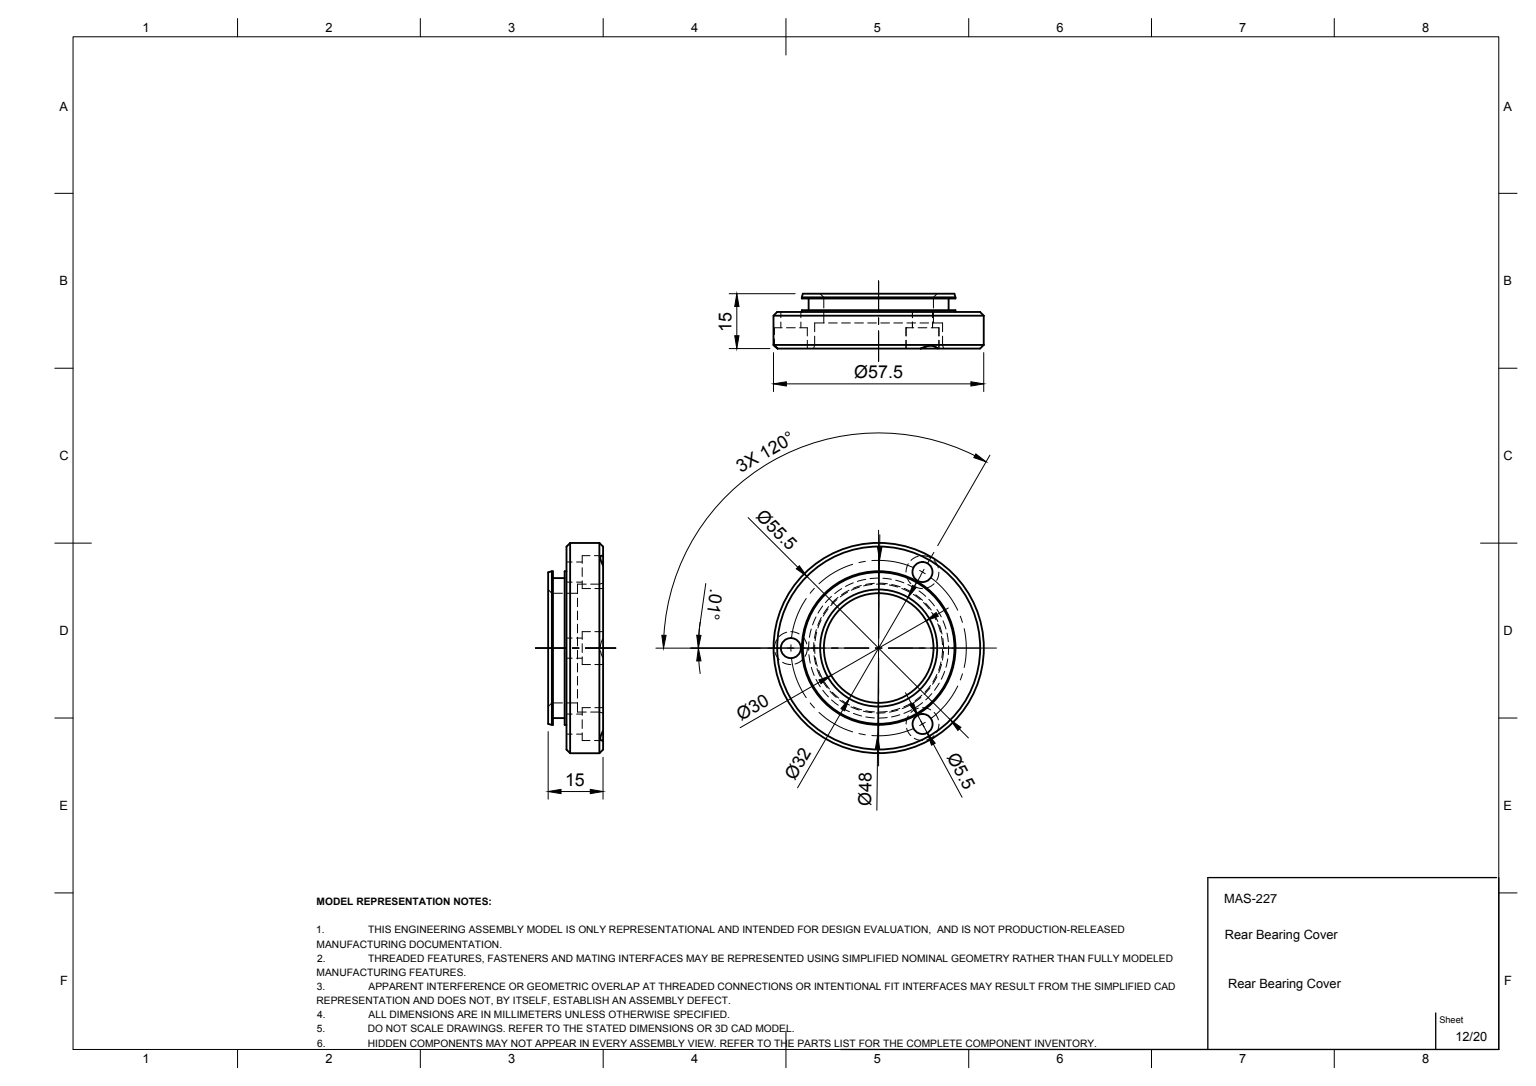
ISO-10303-21;
HEADER;
FILE_DESCRIPTION (('STEP AP214'),
    '1' );
FILE_NAME ( 'Rear Bearing Cover.step', '2026-10-06T08:24:41', ( '' ), ( '' ), 'STEP AP214', 'Unspecified', '' );
FILE_SCHEMA (( 'AUTOMOTIVE_DESIGN' ));
ENDSEC;
DATA;
#7=DIRECTION ( 'NONE',  ( -1.000000000000000000, 0.000000000000000000, 0.000000000000000000 ) ) ;
#24=ORIENTED_EDGE ( 'NONE', *, *, #27873, .F. ) ;
#69=DIRECTION ( 'NONE',  ( 1.000000000000000000, 0.000000000000000000, 0.000000000000000000 ) ) ;
#80=EDGE_LOOP ( 'NONE', ( #10881, #7158 ) ) ;
#89=DIRECTION ( 'NONE',  ( 0.000000000000000000, -1.000000000000000000, 0.000000000000000000 ) ) ;
#102=DIRECTION ( 'NONE',  ( -1.000000000000000000, 0.000000000000000000, 0.000000000000000000 ) ) ;
#208=CARTESIAN_POINT ( 'NONE',  ( -0.01968503937007897581, -0.8214970631411201429, 0.000000000000000000 ) ) ;
#218=VERTEX_POINT ( 'NONE', #1034 ) ;
#239=EDGE_LOOP ( 'NONE', ( #22677, #15160 ) ) ;
#245=DIRECTION ( 'NONE',  ( -1.000000000000000000, 0.000000000000000000, 0.000000000000000000 ) ) ;
#268=ORIENTED_EDGE ( 'NONE', *, *, #11086, .F. ) ;
#315=FACE_OUTER_BOUND ( 'NONE', #4485, .T. ) ;
#445=VECTOR ( 'NONE', #20789, 39.37007874015748854 ) ;
#447=FACE_OUTER_BOUND ( 'NONE', #2356, .T. ) ;
#465=DIRECTION ( 'NONE',  ( 1.000000000000000000, 0.000000000000000000, 0.000000000000000000 ) ) ;
#470=CIRCLE ( 'NONE', #7684, 0.6889763779527560139 ) ;
#587=CIRCLE ( 'NONE', #3254, 0.8267716535433071723 ) ;
#589=ORIENTED_EDGE ( 'NONE', *, *, #19290, .F. ) ;
#648=CARTESIAN_POINT ( 'NONE',  ( -0.01968503937007897581, 0.8214970631411201429, 1.006043748884723849E-16 ) ) ;
#653=DIRECTION ( 'NONE',  ( 0.000000000000000000, -1.000000000000000000, 0.000000000000000000 ) ) ;
#671=DIRECTION ( 'NONE',  ( 0.000000000000000000, -1.000000000000000000, 0.000000000000000000 ) ) ;
#813=DIRECTION ( 'NONE',  ( 1.000000000000000000, 0.000000000000000000, 0.000000000000000000 ) ) ;
#828=ORIENTED_EDGE ( 'NONE', *, *, #19338, .F. ) ;
#844=CIRCLE ( 'NONE', #25418, 0.1771653543307086798 ) ;
#853=CARTESIAN_POINT ( 'NONE',  ( -0.3661417322834645272, -0.4724409448818898127, -0.8182917201112815953 ) ) ;
#863=CYLINDRICAL_SURFACE ( 'NONE', #6726, 0.7539370078740157410 ) ;
#903=ORIENTED_EDGE ( 'NONE', *, *, #16753, .T. ) ;
#912=DIRECTION ( 'NONE',  ( 1.000000000000000000, 0.000000000000000000, 0.000000000000000000 ) ) ;
#919=DIRECTION ( 'NONE',  ( 1.000000000000000000, 0.000000000000000000, 0.000000000000000000 ) ) ;
#989=CARTESIAN_POINT ( 'NONE',  ( -0.3149606299212598381, 0.000000000000000000, 0.000000000000000000 ) ) ;
#1005=ORIENTED_EDGE ( 'NONE', *, *, #22105, .F. ) ;
#1030=CIRCLE ( 'NONE', #19050, 0.8162224727389330026 ) ;
#1034=CARTESIAN_POINT ( 'NONE',  ( -0.5905511811023621549, 0.6995255587508188988, 8.566717364459539934E-17 ) ) ;
#1053=CIRCLE ( 'NONE', #16846, 0.1082677165354330312 ) ;
#1091=ORIENTED_EDGE ( 'NONE', *, *, #9443, .F. ) ;
#1121=ORIENTED_EDGE ( 'NONE', *, *, #6645, .T. ) ;
#1143=CIRCLE ( 'NONE', #10607, 0.1082677165354330312 ) ;
#1159=CARTESIAN_POINT ( 'NONE',  ( -0.1968503937007874127, 0.000000000000000000, 0.000000000000000000 ) ) ;
#1234=DIRECTION ( 'NONE',  ( -1.000000000000000000, 0.000000000000000000, 0.000000000000000000 ) ) ;
#1254=DIRECTION ( 'NONE',  ( 1.000000000000000000, 0.000000000000000000, 0.000000000000000000 ) ) ;
#1287=CARTESIAN_POINT ( 'NONE',  ( -0.1771653543307086520, 0.000000000000000000, 0.000000000000000000 ) ) ;
#1312=SURFACE_SIDE_STYLE ('',( #11903 ) ) ;
#1384=CARTESIAN_POINT ( 'NONE',  ( 2.664928230027803213, 0.9448818897637796255, -1.639108661417322569E-17 ) ) ;
#1398=CARTESIAN_POINT ( 'NONE',  ( -0.5811915241081616612, -0.4724399524670138684, 0.9954595399565421276 ) ) ;
#1402=PLANE ( 'NONE',  #15530 ) ;
#1403=AXIS2_PLACEMENT_3D ( 'NONE', #19008, #6721, #21281 ) ;
#1430=DIRECTION ( 'NONE',  ( 0.000000000000000000, -1.000000000000000000, 0.000000000000000000 ) ) ;
#1484=CIRCLE ( 'NONE', #8268, 0.6299212598425196763 ) ;
#1488=DIRECTION ( 'NONE',  ( 0.000000000000000000, 1.000000000000000000, 0.000000000000000000 ) ) ;
#1496=FACE_OUTER_BOUND ( 'NONE', #23490, .T. ) ;
#1544=ORIENTED_EDGE ( 'NONE', *, *, #11001, .F. ) ;
#1548=FACE_OUTER_BOUND ( 'NONE', #9863, .T. ) ;
#1550=DIRECTION ( 'NONE',  ( -1.000000000000000000, 0.000000000000000000, 0.000000000000000000 ) ) ;
#1579=CARTESIAN_POINT ( 'NONE',  ( -0.5708661417322835607, 0.000000000000000000, 0.000000000000000000 ) ) ;
#1596=CARTESIAN_POINT ( 'NONE',  ( -0.5609636804891235951, -0.5548708868579311781, 0.9753553170056504795 ) ) ;
#1599=CARTESIAN_POINT ( 'NONE',  ( -0.5622642684307268546, -0.5391005349161613891, -0.9826765462749343927 ) ) ;
#1600=FACE_OUTER_BOUND ( 'NONE', #23729, .T. ) ;
#1624=PLANE ( 'NONE',  #18273 ) ;
#1625=FACE_BOUND ( 'NONE', #12857, .T. ) ;
#1645=FACE_OUTER_BOUND ( 'NONE', #3746, .T. ) ;
#1655=CIRCLE ( 'NONE', #3429, 0.1771653543307086798 ) ;
#1676=AXIS2_PLACEMENT_3D ( 'NONE', #17009, #8543, #17159 ) ;
#1738=CARTESIAN_POINT ( 'NONE',  ( -0.5616991426751372085, -0.5770957586701074282, 0.9615147744167586996 ) ) ;
#1763=FACE_OUTER_BOUND ( 'NONE', #3029, .T. ) ;
#1767=CONICAL_SURFACE ( 'NONE', #12147, 0.6102362204724409711, 0.7853981625000032718 ) ;
#1771=PLANE ( 'NONE',  #16654 ) ;
#1773=DIRECTION ( 'NONE',  ( 0.000000000000000000, 0.000000000000000000, 1.000000000000000000 ) ) ;
#1855=DIRECTION ( 'NONE',  ( -1.000000000000000000, 0.000000000000000000, 0.000000000000000000 ) ) ;
#1882=PRODUCT_DEFINITION ( 'UNKNOWN', '', #26496, #17018 ) ;
#1918=DIRECTION ( 'NONE',  ( -1.000000000000000000, 0.000000000000000000, 0.000000000000000000 ) ) ;
#1935=VERTEX_POINT ( 'NONE', #20033 ) ;
#1979=DIRECTION ( 'NONE',  ( 1.000000000000000000, 0.000000000000000000, 0.000000000000000000 ) ) ;
#1980=AXIS2_PLACEMENT_3D ( 'NONE', #7829, #5567, #26603 ) ;
#1995=ORIENTED_EDGE ( 'NONE', *, *, #12248, .F. ) ;
#2026=LINE ( 'NONE', #12899, #6921 ) ;
#2044=DIRECTION ( 'NONE',  ( 1.000000000000000000, 0.000000000000000000, 0.000000000000000000 ) ) ;
#2049=VERTEX_POINT ( 'NONE', #7046 ) ;
#2062=DIRECTION ( 'NONE',  ( 1.000000000000000000, 0.000000000000000000, 0.000000000000000000 ) ) ;
#2064=PLANE ( 'NONE',  #7665 ) ;
#2079=CARTESIAN_POINT ( 'NONE',  ( -0.5708661417322835607, 1.112204724409448842, -1.362057955744595713E-16 ) ) ;
#2103=EDGE_LOOP ( 'NONE', ( #16313, #11756, #24, #10103 ) ) ;
#2107=CARTESIAN_POINT ( 'NONE',  ( -0.5681815575442429322, 1.113574658101619930, 0.05417226358512977624 ) ) ;
#2114=CARTESIAN_POINT ( 'NONE',  ( -0.05118110236220472370, 0.000000000000000000, 0.000000000000000000 ) ) ;
#2165=ORIENTED_EDGE ( 'NONE', *, *, #5688, .F. ) ;
#2201=FACE_BOUND ( 'NONE', #13567, .T. ) ;
#2222=VERTEX_POINT ( 'NONE', #5776 ) ;
#2224=DIRECTION ( 'NONE',  ( -1.000000000000000000, 0.000000000000000000, 0.000000000000000000 ) ) ;
#2253=DIRECTION ( 'NONE',  ( 1.000000000000000000, 0.000000000000000000, 0.000000000000000000 ) ) ;
#2285=ORIENTED_EDGE ( 'NONE', *, *, #21450, .F. ) ;
#2287=ADVANCED_FACE ( 'NONE', ( #12776 ), #25780, .T. ) ;
#2301=DIRECTION ( 'NONE',  ( 0.000000000000000000, 0.000000000000000000, 1.000000000000000000 ) ) ;
#2302=ADVANCED_FACE ( 'NONE', ( #27767, #15193 ), #1624, .T. ) ;
#2356=EDGE_LOOP ( 'NONE', ( #13538, #26483, #11394, #8210 ) ) ;
#2363=CARTESIAN_POINT ( 'NONE',  ( -0.1968503937007874127, -0.4724409448818898127, 0.8182917201112815953 ) ) ;
#2369=VECTOR ( 'NONE', #13146, 39.37007874015748143 ) ;
#2377=ORIENTED_EDGE ( 'NONE', *, *, #27274, .F. ) ;
#2380=CARTESIAN_POINT ( 'NONE',  ( -2.185478346456693112E-16, 0.000000000000000000, 0.000000000000000000 ) ) ;
#2382=VECTOR ( 'NONE', #13266, 39.37007874015748143 ) ;
#2412=CARTESIAN_POINT ( 'NONE',  ( -0.5511811023622047445, -0.6889763779527560139, 8.437527159479796553E-17 ) ) ;
#2423=DIRECTION ( 'NONE',  ( 1.000000000000000000, 0.000000000000000000, 0.000000000000000000 ) ) ;
#2424=ORIENTED_EDGE ( 'NONE', *, *, #27873, .T. ) ;
#2434=VECTOR ( 'NONE', #8777, 39.37007874015748143 ) ;
#2438=CARTESIAN_POINT ( 'NONE',  ( -0.5708661417322835607, -0.6942509683549429322, 0.000000000000000000 ) ) ;
#2469=CARTESIAN_POINT ( 'NONE',  ( -0.02559055118110236185, 0.000000000000000000, 0.000000000000000000 ) ) ;
#2512=CARTESIAN_POINT ( 'NONE',  ( -0.3661417322834645272, 0.9448818897637796255, -1.639108661417322569E-17 ) ) ;
#2523=CARTESIAN_POINT ( 'NONE',  ( -0.05118110236220472370, 0.7903543307086614567, 0.000000000000000000 ) ) ;
#2528=CARTESIAN_POINT ( 'NONE',  ( -0.1141732283464566844, 0.7539370078740157410, 0.000000000000000000 ) ) ;
#2549=VECTOR ( 'NONE', #10663, 39.37007874015748143 ) ;
#2605=AXIS2_PLACEMENT_3D ( 'NONE', #9872, #10429, #27399 ) ;
#2610=AXIS2_PLACEMENT_3D ( 'NONE', #8395, #23235, #3870 ) ;
#2643=ORIENTED_EDGE ( 'NONE', *, *, #3133, .T. ) ;
#2656=AXIS2_PLACEMENT_3D ( 'NONE', #9060, #23786, #89 ) ;
#2687=DIRECTION ( 'NONE',  ( 0.000000000000000000, -1.000000000000000000, 0.000000000000000000 ) ) ;
#2728=ADVANCED_FACE ( 'NONE', ( #4189 ), #21424, .T. ) ;
#2758=EDGE_LOOP ( 'NONE', ( #12853, #9072, #23845, #6887 ) ) ;
#2760=EDGE_CURVE ( 'NONE', #13081, #6094, #26969, .T. ) ;
#2826=VECTOR ( 'NONE', #2224, 39.37007874015748143 ) ;
#2839=CARTESIAN_POINT ( 'NONE',  ( -0.05118110236220472370, 0.8267716535433071723, 0.000000000000000000 ) ) ;
#2859=CYLINDRICAL_SURFACE ( 'NONE', #19118, 0.8267716535433071723 ) ;
#2860=VECTOR ( 'NONE', #11180, 39.37007874015748143 ) ;
#2904=CONICAL_SURFACE ( 'NONE', #12415, 1.112204724409448842, 0.7853981625000011624 ) ;
#2954=CYLINDRICAL_SURFACE ( 'NONE', #14208, 0.1771653543307086798 ) ;
#2963=ORIENTED_EDGE ( 'NONE', *, *, #26481, .F. ) ;
#3024=CARTESIAN_POINT ( 'NONE',  ( -0.03937007874015747977, 0.000000000000000000, 0.000000000000000000 ) ) ;
#3027=VERTEX_POINT ( 'NONE', #12489 ) ;
#3029=EDGE_LOOP ( 'NONE', ( #11928, #9052, #17562, #5731, #24652 ) ) ;
#3074=EDGE_CURVE ( 'NONE', #14891, #4135, #23792, .T. ) ;
#3080=AXIS2_PLACEMENT_3D ( 'NONE', #20906, #1550, #16814 ) ;
#3109=EDGE_CURVE ( 'NONE', #9597, #14042, #11187, .T. ) ;
#3124=CARTESIAN_POINT ( 'NONE',  ( -0.4783464566929133688, -0.4724409448818898127, -0.8182917201112815953 ) ) ;
#3133=EDGE_CURVE ( 'NONE', #12001, #8922, #22523, .T. ) ;
#3146=LINE ( 'NONE', #11777, #7662 ) ;
#3178=ORIENTED_EDGE ( 'NONE', *, *, #23388, .T. ) ;
#3232=VERTEX_POINT ( 'NONE', #22378 ) ;
#3239=VERTEX_POINT ( 'NONE', #12065 ) ;
#3254=AXIS2_PLACEMENT_3D ( 'NONE', #4997, #919, #13619 ) ;
#3261=DIRECTION ( 'NONE',  ( -1.000000000000000000, 0.000000000000000000, 0.000000000000000000 ) ) ;
#3278=CARTESIAN_POINT ( 'NONE',  ( -0.3149606299212598381, 0.000000000000000000, 0.000000000000000000 ) ) ;
#3293=VERTEX_POINT ( 'NONE', #9801 ) ;
#3312=CARTESIAN_POINT ( 'NONE',  ( -0.03937007874015747977, 0.000000000000000000, 0.000000000000000000 ) ) ;
#3325=EDGE_CURVE ( 'NONE', #25692, #23663, #26075, .T. ) ;
#3357=EDGE_LOOP ( 'NONE', ( #19208, #4870, #20216, #2165 ) ) ;
#3360=UNCERTAINTY_MEASURE_WITH_UNIT (LENGTH_MEASURE( 1.000000000000000082E-05 ), #12173, 'distance_accuracy_value', 'NONE') ;
#3429=AXIS2_PLACEMENT_3D ( 'NONE', #25649, #6303, #23547 ) ;
#3441=ORIENTED_EDGE ( 'NONE', *, *, #26709, .T. ) ;
#3463=DIRECTION ( 'NONE',  ( 0.000000000000000000, -1.000000000000000000, 0.000000000000000000 ) ) ;
#3495=DIRECTION ( 'NONE',  ( -1.000000000000000000, 0.000000000000000000, 0.000000000000000000 ) ) ;
#3516=VECTOR ( 'NONE', #2253, 39.37007874015748143 ) ;
#3534=CARTESIAN_POINT ( 'NONE',  ( -2.185478346456693112E-16, 0.000000000000000000, 0.000000000000000000 ) ) ;
#3537=VECTOR ( 'NONE', #15870, 39.37007874015748143 ) ;
#3546=AXIS2_PLACEMENT_3D ( 'NONE', #17760, #9267, #5182 ) ;
#3575=SHAPE_REPRESENTATION ( 'Rear Bearing Cover', ( #11588 ), #19278 ) ;
#3610=CARTESIAN_POINT ( 'NONE',  ( -0.05118110236220472370, 0.7539370078740157410, 0.000000000000000000 ) ) ;
#3665=DIRECTION ( 'NONE',  ( 0.000000000000000000, 0.000000000000000000, 1.000000000000000000 ) ) ;
#3681=ORIENTED_EDGE ( 'NONE', *, *, #6118, .F. ) ;
#3697=AXIS2_PLACEMENT_3D ( 'NONE', #11160, #17904, #22309 ) ;
#3714=CARTESIAN_POINT ( 'NONE',  ( -0.5616993144963264850, -0.5770964849842729061, -0.9615141454532954990 ) ) ;
#3728=CONICAL_SURFACE ( 'NONE', #24035, 0.8214970631411201429, 0.2617993875000020898 ) ;
#3746=EDGE_LOOP ( 'NONE', ( #23859, #6534 ) ) ;
#3789=ORIENTED_EDGE ( 'NONE', *, *, #4673, .F. ) ;
#3797=EDGE_CURVE ( 'NONE', #16095, #12969, #16768, .T. ) ;
#3800=DIRECTION ( 'NONE',  ( 0.000000000000000000, 0.000000000000000000, 1.000000000000000000 ) ) ;
#3809=DIRECTION ( 'NONE',  ( -1.000000000000000000, 0.000000000000000000, 0.000000000000000000 ) ) ;
#3819=VERTEX_POINT ( 'NONE', #5474 ) ;
#3835=ORIENTED_EDGE ( 'NONE', *, *, #10679, .F. ) ;
#3863=CARTESIAN_POINT ( 'NONE',  ( -0.5819147541874519769, -0.6280848967520352710, -0.9045786101298314286 ) ) ;
#3870=DIRECTION ( 'NONE',  ( 0.000000000000000000, 0.000000000000000000, 1.000000000000000000 ) ) ;
#3887=DIRECTION ( 'NONE',  ( 0.000000000000000000, 0.000000000000000000, 1.000000000000000000 ) ) ;
#3891=ORIENTED_EDGE ( 'NONE', *, *, #11596, .T. ) ;
#3892=VERTEX_POINT ( 'NONE', #24953 ) ;
#3897=ORIENTED_EDGE ( 'NONE', *, *, #14924, .T. ) ;
#3905=CARTESIAN_POINT ( 'NONE',  ( -0.1574803149606299191, 0.000000000000000000, 0.000000000000000000 ) ) ;
#3936=DIRECTION ( 'NONE',  ( 0.000000000000000000, -1.000000000000000000, 0.000000000000000000 ) ) ;
#3942=CARTESIAN_POINT ( 'NONE',  ( -0.4783464566929133688, 0.9448818897637796255, -1.639108661417322569E-17 ) ) ;
#3951=DIRECTION ( 'NONE',  ( 0.000000000000000000, 0.000000000000000000, 1.000000000000000000 ) ) ;
#3973=CARTESIAN_POINT ( 'NONE',  ( -0.5905511811023621549, -0.6348133144914153148, 0.8891632684400255782 ) ) ;
#4008=ADVANCED_FACE ( 'NONE', ( #11441 ), #20198, .F. ) ;
#4012=CARTESIAN_POINT ( 'NONE',  ( -0.3661417322834645272, 0.9448818897637796255, -0.1771653543307086520 ) ) ;
#4025=EDGE_LOOP ( 'NONE', ( #15939, #13089, #26409, #6919 ) ) ;
#4029=ADVANCED_FACE ( 'NONE', ( #16112 ), #863, .T. ) ;
#4036=DIRECTION ( 'NONE',  ( 0.000000000000000000, 0.000000000000000000, 1.000000000000000000 ) ) ;
#4051=CARTESIAN_POINT ( 'NONE',  ( -2.185478346456693112E-16, -0.6299212598071869396, 0.000000000000000000 ) ) ;
#4082=CARTESIAN_POINT ( 'NONE',  ( -0.4783464566929133688, -0.4724409448818898127, -0.8182917201112815953 ) ) ;
#4099=EDGE_CURVE ( 'NONE', #22689, #27836, #10771, .T. ) ;
#4111=DIRECTION ( 'NONE',  ( 0.000000000000000000, 0.000000000000000000, 1.000000000000000000 ) ) ;
#4127=DIRECTION ( 'NONE',  ( -1.000000000000000000, 0.000000000000000000, 0.000000000000000000 ) ) ;
#4135=VERTEX_POINT ( 'NONE', #20026 ) ;
#4139=CARTESIAN_POINT ( 'NONE',  ( 2.664928230027803213, -0.4724409448818898127, -0.9265594366467145848 ) ) ;
#4146=CARTESIAN_POINT ( 'NONE',  ( -0.5608506285916234901, -0.5625436374635495174, -0.9710811323268585538 ) ) ;
#4164=ORIENTED_EDGE ( 'NONE', *, *, #25217, .F. ) ;
#4189=FACE_OUTER_BOUND ( 'NONE', #17127, .T. ) ;
#4190=FACE_OUTER_BOUND ( 'NONE', #26019, .T. ) ;
#4248=DIRECTION ( 'NONE',  ( 1.000000000000000000, 0.000000000000000000, 0.000000000000000000 ) ) ;
#4275=ORIENTED_EDGE ( 'NONE', *, *, #25762, .T. ) ;
#4285=AXIS2_PLACEMENT_3D ( 'NONE', #25571, #8469, #12703 ) ;
#4293=LINE ( 'NONE', #11400, #12043 ) ;
#4334=EDGE_LOOP ( 'NONE', ( #26514, #26729, #27046, #19687 ) ) ;
#4367=CARTESIAN_POINT ( 'NONE',  ( -0.5810616737516007824, 1.098416878720776424, 0.09031125883555725375 ) ) ;
#4384=ORIENTED_EDGE ( 'NONE', *, *, #25655, .T. ) ;
#4441=CIRCLE ( 'NONE', #14833, 0.6889763779527560139 ) ;
#4447=DIRECTION ( 'NONE',  ( 0.000000000000000000, 0.000000000000000000, 1.000000000000000000 ) ) ;
#4451=ORIENTED_EDGE ( 'NONE', *, *, #4099, .F. ) ;
#4463=CARTESIAN_POINT ( 'NONE',  ( -0.3661417322834645272, -0.4724409448818898127, -0.6411263657805729155 ) ) ;
#4485=EDGE_LOOP ( 'NONE', ( #17552, #1995, #17553, #9444 ) ) ;
#4568=APPLICATION_CONTEXT ( 'automotive_design' ) ;
#4589=DIRECTION ( 'NONE',  ( 0.000000000000000000, -1.000000000000000000, 0.000000000000000000 ) ) ;
#4591=EDGE_CURVE ( 'NONE', #14336, #3819, #14026, .T. ) ;
#4599=DIRECTION ( 'NONE',  ( 1.000000000000000000, 0.000000000000000000, 0.000000000000000000 ) ) ;
#4622=DIRECTION ( 'NONE',  ( -1.000000000000000000, 0.000000000000000000, 0.000000000000000000 ) ) ;
#4650=EDGE_CURVE ( 'NONE', #2222, #5851, #10328, .T. ) ;
#4662=DIRECTION ( 'NONE',  ( 0.000000000000000000, 0.000000000000000000, 1.000000000000000000 ) ) ;
#4665=VECTOR ( 'NONE', #13639, 39.37007874015748854 ) ;
#4673=EDGE_CURVE ( 'NONE', #25416, #22409, #21629, .T. ) ;
#4705=CIRCLE ( 'NONE', #24121, 0.7539370078740157410 ) ;
#4712=CARTESIAN_POINT ( 'NONE',  ( 2.664928230027803213, -0.4724409448818898127, 0.9265594366467145848 ) ) ;
#4751=CIRCLE ( 'NONE', #16056, 0.8267716535433071723 ) ;
#4775=ORIENTED_EDGE ( 'NONE', *, *, #23661, .F. ) ;
#4817=CARTESIAN_POINT ( 'NONE',  ( -0.5905511811023621549, 0.000000000000000000, 0.000000000000000000 ) ) ;
#4870=ORIENTED_EDGE ( 'NONE', *, *, #4591, .T. ) ;
#4878=DIRECTION ( 'NONE',  ( 0.7071067818211385081, 0.7071067805519564153, -8.659560554583433905E-17 ) ) ;
#4906=CARTESIAN_POINT ( 'NONE',  ( -0.5610235350335921467, 1.122047331090474165, 0.009609423978176654876 ) ) ;
#4942=ADVANCED_FACE ( 'NONE', ( #20516 ), #26719, .F. ) ;
#4953=EDGE_LOOP ( 'NONE', ( #14615, #22620 ) ) ;
#4968=EDGE_CURVE ( 'NONE', #6094, #25761, #18367, .T. ) ;
#4997=CARTESIAN_POINT ( 'NONE',  ( -0.05118110236220472370, 0.000000000000000000, 0.000000000000000000 ) ) ;
#5023=VERTEX_POINT ( 'NONE', #2839 ) ;
#5035=AXIS2_PLACEMENT_3D ( 'NONE', #23800, #15468, #4447 ) ;
#5059=ORIENTED_EDGE ( 'NONE', *, *, #16111, .T. ) ;
#5109=CONICAL_SURFACE ( 'NONE', #26758, 0.8214970631411201429, 0.2617993875000020898 ) ;
#5111=CARTESIAN_POINT ( 'NONE',  ( 2.664928230027803213, 0.9448818897637796255, -0.1082677165354330867 ) ) ;
#5162=CARTESIAN_POINT ( 'NONE',  ( -0.5511811023622047445, -1.131889763744194921, 0.000000000000000000 ) ) ;
#5182=DIRECTION ( 'NONE',  ( 0.000000000000000000, 0.000000000000000000, 1.000000000000000000 ) ) ;
#5229=CARTESIAN_POINT ( 'NONE',  ( 0.000000000000000000, 0.000000000000000000, 0.000000000000000000 ) ) ;
#5275=DIRECTION ( 'NONE',  ( 0.000000000000000000, 1.000000000000000000, 0.000000000000000000 ) ) ;
#5283=ORIENTED_EDGE ( 'NONE', *, *, #17027, .F. ) ;
#5327=EDGE_CURVE ( 'NONE', #4135, #218, #13931, .T. ) ;
#5371=CARTESIAN_POINT ( 'NONE',  ( -0.1968503937007874127, -1.092519685039370136, 0.000000000000000000 ) ) ;
#5389=EDGE_LOOP ( 'NONE', ( #10548, #6140, #22300, #27754, #5059, #10387, #9766, #7521 ) ) ;
#5446=AXIS2_PLACEMENT_3D ( 'NONE', #4082, #10991, #26103 ) ;
#5458=EDGE_LOOP ( 'NONE', ( #21728, #2377, #20398, #4775, #12744 ) ) ;
#5474=CARTESIAN_POINT ( 'NONE',  ( -0.3661417322834645272, 0.9448818897637796255, -0.1082677165354330867 ) ) ;
#5493=( NAMED_UNIT ( * ) PLANE_ANGLE_UNIT ( ) SI_UNIT ( $, .RADIAN. ) ) ;
#5511=AXIS2_PLACEMENT_3D ( 'NONE', #8109, #25334, #5997 ) ;
#5530=VERTEX_POINT ( 'NONE', #19268 ) ;
#5538=VERTEX_POINT ( 'NONE', #18305 ) ;
#5554=ORIENTED_EDGE ( 'NONE', *, *, #14924, .F. ) ;
#5561=CIRCLE ( 'NONE', #21360, 0.5905511811023621549 ) ;
#5567=DIRECTION ( 'NONE',  ( -1.000000000000000000, 0.000000000000000000, 0.000000000000000000 ) ) ;
#5578=ORIENTED_EDGE ( 'NONE', *, *, #25900, .T. ) ;
#5616=CARTESIAN_POINT ( 'NONE',  ( -0.03937007874015747977, 0.8267716535433071723, 0.000000000000000000 ) ) ;
#5638=LINE ( 'NONE', #22876, #7955 ) ;
#5645=CARTESIAN_POINT ( 'NONE',  ( -0.3661417322834645272, 0.9448818897637796255, -1.639108661417322569E-17 ) ) ;
#5654=FACE_OUTER_BOUND ( 'NONE', #7739, .T. ) ;
#5688=EDGE_CURVE ( 'NONE', #27195, #3027, #10932, .T. ) ;
#5698=( NAMED_UNIT ( * ) SI_UNIT ( $, .STERADIAN. ) SOLID_ANGLE_UNIT ( ) ) ;
#5712=DIRECTION ( 'NONE',  ( -1.000000000000000000, 0.000000000000000000, 0.000000000000000000 ) ) ;
#5731=ORIENTED_EDGE ( 'NONE', *, *, #16111, .F. ) ;
#5746=ORIENTED_EDGE ( 'NONE', *, *, #16205, .T. ) ;
#5774=ORIENTED_EDGE ( 'NONE', *, *, #27188, .T. ) ;
#5776=CARTESIAN_POINT ( 'NONE',  ( -0.1968503937007874127, 1.092519685039370136, 1.362057955722570717E-16 ) ) ;
#5806=FACE_OUTER_BOUND ( 'NONE', #5458, .T. ) ;
#5850=CARTESIAN_POINT ( 'NONE',  ( -0.5670362563030384440, -0.5142385541158210893, 0.9905098495110491452 ) ) ;
#5851=VERTEX_POINT ( 'NONE', #25843 ) ;
#5890=CARTESIAN_POINT ( 'NONE',  ( -0.1574803149606299191, -0.5905511811023621549, 7.232166136696967594E-17 ) ) ;
#5917=VERTEX_POINT ( 'NONE', #13177 ) ;
#5927=ORIENTED_EDGE ( 'NONE', *, *, #27300, .T. ) ;
#5929=B_SPLINE_CURVE_WITH_KNOTS ( 'NONE', 3,
 ( #13518, #4906, #21606, #17494, #15124, #13253, #15403, #2107, #22014, #4367, #25842 ),
 .UNSPECIFIED., .F., .F.,
 ( 4, 2, 1, 2, 2, 4 ),
 ( 0.5000000000000000000, 0.6250000000000006661, 0.6875000000000007772, 0.7187500000000007772, 0.7500000000000008882, 1.000000000000000000 ),
 .UNSPECIFIED. ) ;
#5931=DIRECTION ( 'NONE',  ( -1.000000000000000000, 0.000000000000000000, 0.000000000000000000 ) ) ;
#5960=ORIENTED_EDGE ( 'NONE', *, *, #24424, .F. ) ;
#5961=DIRECTION ( 'NONE',  ( 1.000000000000000000, 0.000000000000000000, 0.000000000000000000 ) ) ;
#5981=EDGE_CURVE ( 'NONE', #5851, #2049, #6284, .T. ) ;
#5992=CARTESIAN_POINT ( 'NONE',  ( -0.5511811023622047445, 0.6889763779527560139, 0.000000000000000000 ) ) ;
#5995=CARTESIAN_POINT ( 'NONE',  ( -0.5905511811023621549, -0.6348133144914153148, -0.8891632684400255782 ) ) ;
#5997=DIRECTION ( 'NONE',  ( 0.000000000000000000, 0.000000000000000000, 1.000000000000000000 ) ) ;
#6033=DIRECTION ( 'NONE',  ( -1.000000000000000000, 0.000000000000000000, 0.000000000000000000 ) ) ;
#6036=CYLINDRICAL_SURFACE ( 'NONE', #14705, 0.5905511811023621549 ) ;
#6042=CIRCLE ( 'NONE', #21816, 0.8267716535433071723 ) ;
#6084=FACE_BOUND ( 'NONE', #239, .T. ) ;
#6094=VERTEX_POINT ( 'NONE', #26714 ) ;
#6118=EDGE_CURVE ( 'NONE', #12001, #22551, #13472, .T. ) ;
#6140=ORIENTED_EDGE ( 'NONE', *, *, #14071, .T. ) ;
#6143=CARTESIAN_POINT ( 'NONE',  ( -0.5692989725251984545, -0.5056979702041203284, -0.9923584033841372776 ) ) ;
#6144=CARTESIAN_POINT ( 'NONE',  ( -0.03937007874015747977, 0.000000000000000000, 0.000000000000000000 ) ) ;
#6163=EDGE_LOOP ( 'NONE', ( #23262, #25298 ) ) ;
#6193=EDGE_LOOP ( 'NONE', ( #16822, #3789, #19449, #4451, #17611 ) ) ;
#6253=DIRECTION ( 'NONE',  ( -1.000000000000000000, 0.000000000000000000, 0.000000000000000000 ) ) ;
#6278=VERTEX_POINT ( 'NONE', #3610 ) ;
#6284=CIRCLE ( 'NONE', #8533, 1.131889763779527547 ) ;
#6292=CARTESIAN_POINT ( 'NONE',  ( -0.5708661417322835607, -1.112204724409448842, 0.000000000000000000 ) ) ;
#6303=DIRECTION ( 'NONE',  ( -1.000000000000000000, 0.000000000000000000, 0.000000000000000000 ) ) ;
#6317=CARTESIAN_POINT ( 'NONE',  ( -0.5905511811023621549, -0.4526313213353566622, -0.9943460912301791410 ) ) ;
#6325=SHAPE_DEFINITION_REPRESENTATION ( #7998, #3575 ) ;
#6363=CARTESIAN_POINT ( 'NONE',  ( -0.3661417322834645272, -0.4724409448818898127, 0.9265594366467145848 ) ) ;
#6390=EDGE_LOOP ( 'NONE', ( #20404, #3441 ) ) ;
#6397=ADVANCED_FACE ( 'NONE', ( #2201, #1645 ), #2064, .T. ) ;
#6409=FACE_OUTER_BOUND ( 'NONE', #7791, .T. ) ;
#6412=ORIENTED_EDGE ( 'NONE', *, *, #4099, .T. ) ;
#6433=VECTOR ( 'NONE', #16014, 39.37007874015748143 ) ;
#6448=EDGE_CURVE ( 'NONE', #14336, #27195, #10811, .T. ) ;
#6461=CARTESIAN_POINT ( 'NONE',  ( -0.4527559055118110520, 0.000000000000000000, 0.000000000000000000 ) ) ;
#6484=ORIENTED_EDGE ( 'NONE', *, *, #24237, .T. ) ;
#6534=ORIENTED_EDGE ( 'NONE', *, *, #26548, .F. ) ;
#6576=DIRECTION ( 'NONE',  ( 1.000000000000000000, 0.000000000000000000, 0.000000000000000000 ) ) ;
#6618=LINE ( 'NONE', #26362, #2826 ) ;
#6645=EDGE_CURVE ( 'NONE', #19029, #17602, #17988, .T. ) ;
#6649=CARTESIAN_POINT ( 'NONE',  ( -0.5736786984127190125, 1.107101695597654922, -0.07148403028362050604 ) ) ;
#6661=CARTESIAN_POINT ( 'NONE',  ( -0.1771653543307086520, -0.8267716535433071723, 1.012503259137575512E-16 ) ) ;
#6664=DIRECTION ( 'NONE',  ( 0.000000000000000000, 0.000000000000000000, 1.000000000000000000 ) ) ;
#6684=VECTOR ( 'NONE', #27612, 39.37007874015748854 ) ;
#6706=LINE ( 'NONE', #6292, #13874 ) ;
#6717=CARTESIAN_POINT ( 'NONE',  ( -0.1771653543307086520, 0.7903543307086614567, 0.000000000000000000 ) ) ;
#6721=DIRECTION ( 'NONE',  ( 1.000000000000000000, 0.000000000000000000, 0.000000000000000000 ) ) ;
#6726=AXIS2_PLACEMENT_3D ( 'NONE', #9448, #20346, #20483 ) ;
#6744=DIRECTION ( 'NONE',  ( 0.000000000000000000, 1.000000000000000000, 0.000000000000000000 ) ) ;
#6757=LINE ( 'NONE', #19739, #18628 ) ;
#6758=EDGE_LOOP ( 'NONE', ( #7160, #14997 ) ) ;
#6791=( GEOMETRIC_REPRESENTATION_CONTEXT ( 3 ) GLOBAL_UNCERTAINTY_ASSIGNED_CONTEXT ( ( #3360 ) ) GLOBAL_UNIT_ASSIGNED_CONTEXT ( ( #12173, #16005, #5698 ) ) REPRESENTATION_CONTEXT ( 'NONE', 'WORKASPACE' ) ) ;
#6800=CARTESIAN_POINT ( 'NONE',  ( -0.1968503937007874127, 0.000000000000000000, 0.000000000000000000 ) ) ;
#6815=CARTESIAN_POINT ( 'NONE',  ( -2.185478346456693112E-16, 0.000000000000000000, 0.000000000000000000 ) ) ;
#6842=CARTESIAN_POINT ( 'NONE',  ( -0.5905511811023621549, -0.6348133144914153148, -0.8891632684400255782 ) ) ;
#6851=ORIENTED_EDGE ( 'NONE', *, *, #4968, .F. ) ;
#6855=CARTESIAN_POINT ( 'NONE',  ( -0.3661417322834645272, -0.4724409448818898127, -0.9265594366467145848 ) ) ;
#6883=LINE ( 'NONE', #11521, #4665 ) ;
#6887=ORIENTED_EDGE ( 'NONE', *, *, #7653, .T. ) ;
#6906=ADVANCED_FACE ( 'NONE', ( #20892 ), #14709, .F. ) ;
#6919=ORIENTED_EDGE ( 'NONE', *, *, #11831, .T. ) ;
#6921=VECTOR ( 'NONE', #8527, 39.37007874015748143 ) ;
#6926=AXIS2_PLACEMENT_3D ( 'NONE', #1384, #15935, #9718 ) ;
#6929=DIRECTION ( 'NONE',  ( 0.000000000000000000, 0.000000000000000000, 1.000000000000000000 ) ) ;
#6948=LINE ( 'NONE', #208, #2434 ) ;
#6992=ORIENTED_EDGE ( 'NONE', *, *, #21821, .T. ) ;
#7001=DIRECTION ( 'NONE',  ( 1.000000000000000000, 0.000000000000000000, 0.000000000000000000 ) ) ;
#7019=CARTESIAN_POINT ( 'NONE',  ( -0.01968503937007897581, 0.000000000000000000, 0.000000000000000000 ) ) ;
#7022=ORIENTED_EDGE ( 'NONE', *, *, #10581, .F. ) ;
#7046=CARTESIAN_POINT ( 'NONE',  ( -0.2362204724409449064, -1.131889763779527547, 1.386165176200252194E-16 ) ) ;
#7049=CARTESIAN_POINT ( 'NONE',  ( -0.4783464566929133688, -0.4724409448818898127, 0.6411263657805729155 ) ) ;
#7060=PLANE ( 'NONE',  #20298 ) ;
#7158=ORIENTED_EDGE ( 'NONE', *, *, #18869, .T. ) ;
#7160=ORIENTED_EDGE ( 'NONE', *, *, #17780, .F. ) ;
#7182=CARTESIAN_POINT ( 'NONE',  ( 2.664928230027803213, -0.4724409448818898127, 0.8182917201112815953 ) ) ;
#7192=DIRECTION ( 'NONE',  ( 0.000000000000000000, 0.000000000000000000, 1.000000000000000000 ) ) ;
#7196=DIRECTION ( 'NONE',  ( 1.000000000000000000, 0.000000000000000000, 0.000000000000000000 ) ) ;
#7223=AXIS2_PLACEMENT_3D ( 'NONE', #22839, #6033, #10243 ) ;
#7246=EDGE_LOOP ( 'NONE', ( #18457, #11037, #5960, #13093, #9921 ) ) ;
#7249=ORIENTED_EDGE ( 'NONE', *, *, #17017, .F. ) ;
#7252=ORIENTED_EDGE ( 'NONE', *, *, #14176, .F. ) ;
#7327=EDGE_LOOP ( 'NONE', ( #8306, #19358, #21764, #1544 ) ) ;
#7329=DIRECTION ( 'NONE',  ( -1.000000000000000000, 0.000000000000000000, 0.000000000000000000 ) ) ;
#7336=LINE ( 'NONE', #11298, #16613 ) ;
#7341=ADVANCED_FACE ( 'NONE', ( #17077 ), #25555, .F. ) ;
#7424=EDGE_LOOP ( 'NONE', ( #12107, #24798 ) ) ;
#7436=FACE_OUTER_BOUND ( 'NONE', #23100, .T. ) ;
#7460=CARTESIAN_POINT ( 'NONE',  ( -0.01968503937007873988, 0.000000000000000000, 0.000000000000000000 ) ) ;
#7471=CARTESIAN_POINT ( 'NONE',  ( -2.185478346456693112E-16, 0.8162224727389330026, 1.006043748880834642E-16 ) ) ;
#7493=ADVANCED_FACE ( 'NONE', ( #18859 ), #15804, .T. ) ;
#7498=FACE_OUTER_BOUND ( 'NONE', #17488, .T. ) ;
#7506=DIRECTION ( 'NONE',  ( -1.000000000000000000, 0.000000000000000000, 0.000000000000000000 ) ) ;
#7521=ORIENTED_EDGE ( 'NONE', *, *, #25217, .T. ) ;
#7524=SURFACE_STYLE_USAGE ( .BOTH. , #1312 ) ;
#7539=DIRECTION ( 'NONE',  ( 1.000000000000000000, 0.000000000000000000, 0.000000000000000000 ) ) ;
#7577=EDGE_CURVE ( 'NONE', #218, #4135, #21242, .T. ) ;
#7582=CARTESIAN_POINT ( 'NONE',  ( -0.5905511811023621549, 0.9448818897637796255, -1.639108661417322569E-17 ) ) ;
#7604=AXIS2_PLACEMENT_3D ( 'NONE', #5645, #22882, #3800 ) ;
#7639=CARTESIAN_POINT ( 'NONE',  ( -0.5905511811023621549, -0.4724409448818898127, -0.6411263657805729155 ) ) ;
#7650=EDGE_LOOP ( 'NONE', ( #7655, #24551, #18992, #5554 ) ) ;
#7653=EDGE_CURVE ( 'NONE', #2049, #5851, #21257, .T. ) ;
#7654=CARTESIAN_POINT ( 'NONE',  ( -0.5811930530674194184, -0.4724394499398544278, -0.9954595798869386725 ) ) ;
#7655=ORIENTED_EDGE ( 'NONE', *, *, #22554, .T. ) ;
#7656=CARTESIAN_POINT ( 'NONE',  ( -0.03937007874015747977, -0.5905511811023621549, 7.232166136696967594E-17 ) ) ;
#7662=VECTOR ( 'NONE', #19254, 39.37007874015748143 ) ;
#7665=AXIS2_PLACEMENT_3D ( 'NONE', #8427, #19153, #21555 ) ;
#7678=ADVANCED_FACE ( 'NONE', ( #8289 ), #21549, .F. ) ;
#7684=AXIS2_PLACEMENT_3D ( 'NONE', #17676, #26296, #11325 ) ;
#7685=DIRECTION ( 'NONE',  ( 0.000000000000000000, 1.000000000000000000, 0.000000000000000000 ) ) ;
#7698=AXIS2_PLACEMENT_3D ( 'NONE', #7723, #16336, #1773 ) ;
#7723=CARTESIAN_POINT ( 'NONE',  ( -0.3661417322834645272, -0.4724409448818898127, -0.8182917201112815953 ) ) ;
#7739=EDGE_LOOP ( 'NONE', ( #17604, #13238, #24828, #22597, #22581, #20039, #8418 ) ) ;
#7762=ORIENTED_EDGE ( 'NONE', *, *, #17027, .T. ) ;
#7783=ORIENTED_EDGE ( 'NONE', *, *, #17921, .F. ) ;
#7791=EDGE_LOOP ( 'NONE', ( #9120, #27812, #8319, #7022 ) ) ;
#7812=FILL_AREA_STYLE_COLOUR ( '', #24372 ) ;
#7829=CARTESIAN_POINT ( 'NONE',  ( 2.664928230027803213, -0.4724409448818898127, -0.8182917201112815953 ) ) ;
#7864=CARTESIAN_POINT ( 'NONE',  ( -0.5905511811023621549, 0.000000000000000000, 0.000000000000000000 ) ) ;
#7923=DIRECTION ( 'NONE',  ( 1.000000000000000000, 0.000000000000000000, 0.000000000000000000 ) ) ;
#7940=DIRECTION ( 'NONE',  ( 1.000000000000000000, 0.000000000000000000, 0.000000000000000000 ) ) ;
#7955=VECTOR ( 'NONE', #3495, 39.37007874015748143 ) ;
#7996=VECTOR ( 'NONE', #18052, 39.37007874015748143 ) ;
#7998=PRODUCT_DEFINITION_SHAPE ( 'NONE', 'NONE',  #1882 ) ;
#8021=AXIS2_PLACEMENT_3D ( 'NONE', #2469, #21286, #13076 ) ;
#8055=CARTESIAN_POINT ( 'NONE',  ( -0.5905511811023621549, -0.4526313213353574949, 0.9943460912301771426 ) ) ;
#8086=AXIS2_PLACEMENT_3D ( 'NONE', #25581, #8757, #4111 ) ;
#8109=CARTESIAN_POINT ( 'NONE',  ( -0.5905511811023621549, -0.4724409448818898127, 0.8182917201112815953 ) ) ;
#8135=FACE_BOUND ( 'NONE', #4953, .T. ) ;
#8142=AXIS2_PLACEMENT_3D ( 'NONE', #9186, #16129, #22476 ) ;
#8154=DIRECTION ( 'NONE',  ( 0.000000000000000000, 0.000000000000000000, 1.000000000000000000 ) ) ;
#8210=ORIENTED_EDGE ( 'NONE', *, *, #5327, .T. ) ;
#8215=DIRECTION ( 'NONE',  ( 0.000000000000000000, -1.000000000000000000, 0.000000000000000000 ) ) ;
#8216=CIRCLE ( 'NONE', #5511, 0.1771653543307086798 ) ;
#8247=DIRECTION ( 'NONE',  ( -1.000000000000000000, 0.000000000000000000, 0.000000000000000000 ) ) ;
#8266=ORIENTED_EDGE ( 'NONE', *, *, #20313, .F. ) ;
#8268=AXIS2_PLACEMENT_3D ( 'NONE', #23977, #15389, #13236 ) ;
#8289=FACE_OUTER_BOUND ( 'NONE', #4025, .T. ) ;
#8297=CARTESIAN_POINT ( 'NONE',  ( -0.5811930530674194184, -0.4724394499398544278, -0.9954595798869386725 ) ) ;
#8305=VECTOR ( 'NONE', #27497, 39.37007874015748143 ) ;
#8306=ORIENTED_EDGE ( 'NONE', *, *, #10189, .F. ) ;
#8319=ORIENTED_EDGE ( 'NONE', *, *, #5981, .T. ) ;
#8327=DIRECTION ( 'NONE',  ( 0.000000000000000000, 0.000000000000000000, 1.000000000000000000 ) ) ;
#8351=ORIENTED_EDGE ( 'NONE', *, *, #2760, .F. ) ;
#8386=CARTESIAN_POINT ( 'NONE',  ( -0.5744829134145985616, -0.4891471943182150173, 0.9948696824535705474 ) ) ;
#8395=CARTESIAN_POINT ( 'NONE',  ( -0.5905511811023621549, 0.9448818897637796255, -1.639108661417322569E-17 ) ) ;
#8412=ORIENTED_EDGE ( 'NONE', *, *, #13636, .F. ) ;
#8418=ORIENTED_EDGE ( 'NONE', *, *, #3109, .F. ) ;
#8427=CARTESIAN_POINT ( 'NONE',  ( -2.158159842519685212E-16, 0.7086614173228346081, 0.000000000000000000 ) ) ;
#8437=PRODUCT_CONTEXT ( 'NONE', #17718, 'mechanical' ) ;
#8469=DIRECTION ( 'NONE',  ( 1.000000000000000000, 0.000000000000000000, 0.000000000000000000 ) ) ;
#8516=EDGE_CURVE ( 'NONE', #16219, #14534, #8216, .T. ) ;
#8519=CIRCLE ( 'NONE', #10330, 0.1771653543307086798 ) ;
#8527=DIRECTION ( 'NONE',  ( 1.000000000000000000, 0.000000000000000000, 0.000000000000000000 ) ) ;
#8533=AXIS2_PLACEMENT_3D ( 'NONE', #11334, #10924, #23794 ) ;
#8539=CIRCLE ( 'NONE', #22532, 1.092519685039370136 ) ;
#8543=DIRECTION ( 'NONE',  ( 1.000000000000000000, 0.000000000000000000, 0.000000000000000000 ) ) ;
#8570=ORIENTED_EDGE ( 'NONE', *, *, #11608, .F. ) ;
#8573=CARTESIAN_POINT ( 'NONE',  ( -0.05118110236220472370, 0.000000000000000000, 0.000000000000000000 ) ) ;
#8582=ORIENTED_EDGE ( 'NONE', *, *, #9817, .F. ) ;
#8617=CARTESIAN_POINT ( 'NONE',  ( -0.5905511811023621549, 1.087444635826771533, -0.1051828227901525498 ) ) ;
#8630=DIRECTION ( 'NONE',  ( 1.000000000000000000, 0.000000000000000000, 0.000000000000000000 ) ) ;
#8640=ORIENTED_EDGE ( 'NONE', *, *, #4968, .T. ) ;
#8742=DIRECTION ( 'NONE',  ( 1.000000000000000000, 0.000000000000000000, 0.000000000000000000 ) ) ;
#8755=DIRECTION ( 'NONE',  ( 0.000000000000000000, 0.000000000000000000, 1.000000000000000000 ) ) ;
#8756=CARTESIAN_POINT ( 'NONE',  ( -0.5714859364026961819, 1.109681230469752089, -0.06506513713611936089 ) ) ;
#8757=DIRECTION ( 'NONE',  ( -1.000000000000000000, 0.000000000000000000, 0.000000000000000000 ) ) ;
#8777=DIRECTION ( 'NONE',  ( -0.9659258263664933786, -0.2588190448135666011, 0.000000000000000000 ) ) ;
#8779=ORIENTED_EDGE ( 'NONE', *, *, #25516, .T. ) ;
#8838=VERTEX_POINT ( 'NONE', #18646 ) ;
#8841=DIRECTION ( 'NONE',  ( 1.000000000000000000, 0.000000000000000000, 0.000000000000000000 ) ) ;
#8845=CYLINDRICAL_SURFACE ( 'NONE', #21731, 0.6889763779527560139 ) ;
#8904=CARTESIAN_POINT ( 'NONE',  ( -0.5905511811023621549, -0.4724409448818898127, 0.8182917201112815953 ) ) ;
#8922=VERTEX_POINT ( 'NONE', #6661 ) ;
#9025=VERTEX_POINT ( 'NONE', #26403 ) ;
#9039=CARTESIAN_POINT ( 'NONE',  ( -0.3661417322834645272, -0.4724409448818898127, 0.6411263657805729155 ) ) ;
#9052=ORIENTED_EDGE ( 'NONE', *, *, #11372, .T. ) ;
#9060=CARTESIAN_POINT ( 'NONE',  ( -0.2165354330708661457, 0.000000000000000000, 0.000000000000000000 ) ) ;
#9072=ORIENTED_EDGE ( 'NONE', *, *, #11218, .T. ) ;
#9116=DIRECTION ( 'NONE',  ( 1.000000000000000000, 0.000000000000000000, 0.000000000000000000 ) ) ;
#9120=ORIENTED_EDGE ( 'NONE', *, *, #21396, .T. ) ;
#9136=ADVANCED_FACE ( 'NONE', ( #447 ), #20865, .F. ) ;
#9186=CARTESIAN_POINT ( 'NONE',  ( -0.1141732283464566844, 0.000000000000000000, 0.000000000000000000 ) ) ;
#9251=CIRCLE ( 'NONE', #24161, 0.8162224727389330026 ) ;
#9267=DIRECTION ( 'NONE',  ( 1.000000000000000000, 0.000000000000000000, 0.000000000000000000 ) ) ;
#9300=CARTESIAN_POINT ( 'NONE',  ( -0.3149606299212598381, 0.6889763779527560139, 0.000000000000000000 ) ) ;
#9344=AXIS2_PLACEMENT_3D ( 'NONE', #26564, #7506, #16132 ) ;
#9387=EDGE_LOOP ( 'NONE', ( #16936, #26294, #3835, #589 ) ) ;
#9430=EDGE_LOOP ( 'NONE', ( #25413, #25440 ) ) ;
#9440=DIRECTION ( 'NONE',  ( 0.000000000000000000, 0.000000000000000000, 1.000000000000000000 ) ) ;
#9443=EDGE_CURVE ( 'NONE', #27816, #5023, #587, .T. ) ;
#9444=ORIENTED_EDGE ( 'NONE', *, *, #14176, .T. ) ;
#9448=CARTESIAN_POINT ( 'NONE',  ( -0.1141732283464566844, 0.000000000000000000, 0.000000000000000000 ) ) ;
#9454=ORIENTED_EDGE ( 'NONE', *, *, #12692, .F. ) ;
#9462=CARTESIAN_POINT ( 'NONE',  ( -0.3937007874015748254, 1.131889763779527547, 0.000000000000000000 ) ) ;
#9484=PRESENTATION_STYLE_ASSIGNMENT (( #7524 ) ) ;
#9489=EDGE_LOOP ( 'NONE', ( #22896, #25049, #12542, #10849 ) ) ;
#9521=FACE_OUTER_BOUND ( 'NONE', #23452, .T. ) ;
#9576=DIRECTION ( 'NONE',  ( 1.000000000000000000, 0.000000000000000000, 0.000000000000000000 ) ) ;
#9597=VERTEX_POINT ( 'NONE', #9941 ) ;
#9600=AXIS2_PLACEMENT_3D ( 'NONE', #23174, #21468, #3951 ) ;
#9606=CYLINDRICAL_SURFACE ( 'NONE', #8142, 0.7539370078740157410 ) ;
#9624=DIRECTION ( 'NONE',  ( -1.000000000000000000, 0.000000000000000000, 0.000000000000000000 ) ) ;
#9625=VECTOR ( 'NONE', #27184, 39.37007874015748143 ) ;
#9685=DIRECTION ( 'NONE',  ( -1.000000000000000000, 0.000000000000000000, 0.000000000000000000 ) ) ;
#9718=DIRECTION ( 'NONE',  ( 0.000000000000000000, 0.000000000000000000, 1.000000000000000000 ) ) ;
#9735=EDGE_CURVE ( 'NONE', #3239, #5530, #17284, .T. ) ;
#9751=ORIENTED_EDGE ( 'NONE', *, *, #20623, .T. ) ;
#9753=AXIS2_PLACEMENT_3D ( 'NONE', #1287, #20777, #18207 ) ;
#9766=ORIENTED_EDGE ( 'NONE', *, *, #22105, .T. ) ;
#9786=CARTESIAN_POINT ( 'NONE',  ( -0.3661417322834645272, -0.4724409448818898127, -0.9954570744419902750 ) ) ;
#9801=CARTESIAN_POINT ( 'NONE',  ( -0.1968503937007874127, -0.4724409448818898127, 0.7100240035758484947 ) ) ;
#9817=EDGE_CURVE ( 'NONE', #27816, #22411, #2026, .T. ) ;
#9846=DIRECTION ( 'NONE',  ( -1.000000000000000000, 0.000000000000000000, 0.000000000000000000 ) ) ;
#9863=EDGE_LOOP ( 'NONE', ( #27140, #14100, #2285, #15497, #2424, #11097, #18670, #6412, #3178, #8412, #22798 ) ) ;
#9872=CARTESIAN_POINT ( 'NONE',  ( -0.3149606299212598381, 0.000000000000000000, 0.000000000000000000 ) ) ;
#9921=ORIENTED_EDGE ( 'NONE', *, *, #13543, .F. ) ;
#9938=CARTESIAN_POINT ( 'NONE',  ( -0.1870078740157480324, -0.8267716535433071723, 1.012503259137575512E-16 ) ) ;
#9941=CARTESIAN_POINT ( 'NONE',  ( -0.5905511811023621549, 0.9448818897637796255, -0.1771653543307086520 ) ) ;
#9957=CIRCLE ( 'NONE', #14507, 0.7539370078740157410 ) ;
#9985=DIRECTION ( 'NONE',  ( 1.000000000000000000, 0.000000000000000000, 0.000000000000000000 ) ) ;
#10005=AXIS2_PLACEMENT_3D ( 'NONE', #18643, #5961, #8215 ) ;
#10020=CARTESIAN_POINT ( 'NONE',  ( -0.5905511811023621549, 0.9448818897637796255, 0.1771653543307086520 ) ) ;
#10023=CARTESIAN_POINT ( 'NONE',  ( -0.5905511811023621549, 0.9104330708661417804, 0.000000000000000000 ) ) ;
#10034=VERTEX_POINT ( 'NONE', #7654 ) ;
#10089=ORIENTED_EDGE ( 'NONE', *, *, #6118, .T. ) ;
#10103=ORIENTED_EDGE ( 'NONE', *, *, #11571, .F. ) ;
#10140=CIRCLE ( 'NONE', #27761, 0.6299212598425196763 ) ;
#10153=AXIS2_PLACEMENT_3D ( 'NONE', #4817, #465, #23649 ) ;
#10189=EDGE_CURVE ( 'NONE', #3293, #21048, #1053, .T. ) ;
#10191=CIRCLE ( 'NONE', #20579, 0.7539370078740157410 ) ;
#10200=CARTESIAN_POINT ( 'NONE',  ( -0.5608505875055256329, -0.5625442442700501200, 0.9710808210050355660 ) ) ;
#10203=CARTESIAN_POINT ( 'NONE',  ( -0.5634519861469524660, -0.5309697779850665045, -0.9857434533500372131 ) ) ;
#10204=DIRECTION ( 'NONE',  ( -1.000000000000000000, 0.000000000000000000, 0.000000000000000000 ) ) ;
#10221=VERTEX_POINT ( 'NONE', #23060 ) ;
#10242=DIRECTION ( 'NONE',  ( 0.000000000000000000, -1.000000000000000000, 0.000000000000000000 ) ) ;
#10243=DIRECTION ( 'NONE',  ( 0.000000000000000000, -1.000000000000000000, 0.000000000000000000 ) ) ;
#10255=AXIS2_PLACEMENT_3D ( 'NONE', #17455, #2062, #10673 ) ;
#10280=AXIS2_PLACEMENT_3D ( 'NONE', #7582, #813, #22696 ) ;
#10328=LINE ( 'NONE', #12164, #445 ) ;
#10330=AXIS2_PLACEMENT_3D ( 'NONE', #8904, #8630, #4662 ) ;
#10349=CARTESIAN_POINT ( 'NONE',  ( -0.5819142500240400695, -0.6280845039713092159, 0.9045795100218007034 ) ) ;
#10375=CARTESIAN_POINT ( 'NONE',  ( -0.3661417322834645272, -0.4724409448818898127, 0.8182917201112815953 ) ) ;
#10387=ORIENTED_EDGE ( 'NONE', *, *, #15270, .T. ) ;
#10421=CARTESIAN_POINT ( 'NONE',  ( -0.1968503937007874127, 0.9448818897637796255, 0.1082677165354330451 ) ) ;
#10429=DIRECTION ( 'NONE',  ( 1.000000000000000000, 0.000000000000000000, 0.000000000000000000 ) ) ;
#10498=ORIENTED_EDGE ( 'NONE', *, *, #4673, .T. ) ;
#10532=B_SPLINE_CURVE_WITH_KNOTS ( 'NONE', 3,
 ( #5995, #3863, #14479, #12335, #23086, #21096, #3714, #4146, #20954, #1599, #10203, #16871, #25480, #6143, #14774, #23379, #25326, #14902 ),
 .UNSPECIFIED., .F., .F.,
 ( 4, 2, 2, 2, 2, 2, 2, 2, 4 ),
 ( 0.000000000000000000, 0.2275410946275231994, 0.3413116419412837166, 0.4550821892550442893, 0.5688527365688048620, 0.6826232838825654348, 0.7395085575394457766, 0.7963938311963262295, 0.9101643785100869133 ),
 .UNSPECIFIED. ) ;
#10548=ORIENTED_EDGE ( 'NONE', *, *, #21821, .F. ) ;
#10557=EDGE_LOOP ( 'NONE', ( #13332, #22184, #11915, #27760 ) ) ;
#10581=EDGE_CURVE ( 'NONE', #13772, #2049, #6883, .T. ) ;
#10607=AXIS2_PLACEMENT_3D ( 'NONE', #853, #20056, #9440 ) ;
#10657=CYLINDRICAL_SURFACE ( 'NONE', #22699, 0.1771653543307086798 ) ;
#10663=DIRECTION ( 'NONE',  ( 1.000000000000000000, 0.000000000000000000, 0.000000000000000000 ) ) ;
#10673=DIRECTION ( 'NONE',  ( 0.000000000000000000, 1.000000000000000000, 0.000000000000000000 ) ) ;
#10675=DIRECTION ( 'NONE',  ( 0.000000000000000000, -1.000000000000000000, 0.000000000000000000 ) ) ;
#10679=EDGE_CURVE ( 'NONE', #14218, #22411, #6042, .T. ) ;
#10741=DIRECTION ( 'NONE',  ( 0.000000000000000000, 1.000000000000000000, 0.000000000000000000 ) ) ;
#10771=CIRCLE ( 'NONE', #3546, 0.1771653543307086798 ) ;
#10811=CIRCLE ( 'NONE', #19382, 0.1082677165354330728 ) ;
#10849=ORIENTED_EDGE ( 'NONE', *, *, #3074, .F. ) ;
#10866=ORIENTED_EDGE ( 'NONE', *, *, #13914, .T. ) ;
#10874=DIRECTION ( 'NONE',  ( 1.000000000000000000, 0.000000000000000000, 0.000000000000000000 ) ) ;
#10881=ORIENTED_EDGE ( 'NONE', *, *, #17918, .T. ) ;
#10893=DIRECTION ( 'NONE',  ( 1.000000000000000000, 0.000000000000000000, 0.000000000000000000 ) ) ;
#10924=DIRECTION ( 'NONE',  ( 1.000000000000000000, 0.000000000000000000, 0.000000000000000000 ) ) ;
#10932=LINE ( 'NONE', #13326, #13023 ) ;
#10947=ORIENTED_EDGE ( 'NONE', *, *, #11730, .T. ) ;
#10991=DIRECTION ( 'NONE',  ( -1.000000000000000000, 0.000000000000000000, 0.000000000000000000 ) ) ;
#11001=EDGE_CURVE ( 'NONE', #21048, #11355, #15476, .T. ) ;
#11016=CARTESIAN_POINT ( 'NONE',  ( -0.3149606299212598381, 0.6397637795275591399, 0.000000000000000000 ) ) ;
#11018=DIRECTION ( 'NONE',  ( 0.000000000000000000, -1.000000000000000000, 0.000000000000000000 ) ) ;
#11032=CARTESIAN_POINT ( 'NONE',  ( -0.3149606299212598381, -0.6889763779527560139, 8.437527159479796553E-17 ) ) ;
#11037=ORIENTED_EDGE ( 'NONE', *, *, #27734, .T. ) ;
#11086=EDGE_CURVE ( 'NONE', #14891, #16095, #21779, .T. ) ;
#11095=FACE_OUTER_BOUND ( 'NONE', #5389, .T. ) ;
#11097=ORIENTED_EDGE ( 'NONE', *, *, #3109, .T. ) ;
#11100=CIRCLE ( 'NONE', #18291, 0.1082677165354330312 ) ;
#11143=CYLINDRICAL_SURFACE ( 'NONE', #23914, 0.1082677165354330312 ) ;
#11160=CARTESIAN_POINT ( 'NONE',  ( -0.5708661417322835607, 0.000000000000000000, 0.000000000000000000 ) ) ;
#11180=DIRECTION ( 'NONE',  ( -1.000000000000000000, 0.000000000000000000, 0.000000000000000000 ) ) ;
#11187=CIRCLE ( 'NONE', #10280, 0.1771653543307086520 ) ;
#11218=EDGE_CURVE ( 'NONE', #2222, #13772, #16376, .T. ) ;
#11289=DIRECTION ( 'NONE',  ( -1.000000000000000000, 0.000000000000000000, 0.000000000000000000 ) ) ;
#11294=CARTESIAN_POINT ( 'NONE',  ( -0.3661417322834645272, -0.4724409448818898127, -0.8182917201112815953 ) ) ;
#11298=CARTESIAN_POINT ( 'NONE',  ( -0.1870078740157480324, 0.8267716535433071723, 0.000000000000000000 ) ) ;
#11312=AXIS2_PLACEMENT_3D ( 'NONE', #25946, #7, #13487 ) ;
#11325=DIRECTION ( 'NONE',  ( 0.000000000000000000, 1.000000000000000000, 0.000000000000000000 ) ) ;
#11334=CARTESIAN_POINT ( 'NONE',  ( -0.2362204724409449064, 0.000000000000000000, 0.000000000000000000 ) ) ;
#11337=EDGE_LOOP ( 'NONE', ( #268, #17619, #23146, #22248 ) ) ;
#11355=VERTEX_POINT ( 'NONE', #6363 ) ;
#11372=EDGE_CURVE ( 'NONE', #19029, #16219, #19485, .T. ) ;
#11390=CONICAL_SURFACE ( 'NONE', #13202, 0.6942509683549429322, 0.2617993875000015902 ) ;
#11394=ORIENTED_EDGE ( 'NONE', *, *, #3074, .T. ) ;
#11400=CARTESIAN_POINT ( 'NONE',  ( -0.02559055118110236185, 0.8267716535433071723, 0.000000000000000000 ) ) ;
#11405=ADVANCED_FACE ( 'NONE', ( #1763 ), #10657, .F. ) ;
#11441=FACE_OUTER_BOUND ( 'NONE', #4334, .T. ) ;
#11466=CARTESIAN_POINT ( 'NONE',  ( -0.3661417322834645272, 0.9448818897637796255, 0.1771653543307086520 ) ) ;
#11475=DIRECTION ( 'NONE',  ( 1.000000000000000000, 0.000000000000000000, 0.000000000000000000 ) ) ;
#11495=LINE ( 'NONE', #20674, #3537 ) ;
#11521=CARTESIAN_POINT ( 'NONE',  ( -0.2165354330708661457, -1.112204724409448842, 0.000000000000000000 ) ) ;
#11571=EDGE_CURVE ( 'NONE', #18321, #23663, #6618, .T. ) ;
#11588=AXIS2_PLACEMENT_3D ( 'NONE', #5229, #3665, #7923 ) ;
#11596=EDGE_CURVE ( 'NONE', #11793, #2049, #6757, .T. ) ;
#11608=EDGE_CURVE ( 'NONE', #5530, #18462, #1484, .T. ) ;
#11661=AXIS2_PLACEMENT_3D ( 'NONE', #18004, #26371, #671 ) ;
#11686=VECTOR ( 'NONE', #3261, 39.37007874015748143 ) ;
#11730=EDGE_CURVE ( 'NONE', #3239, #25537, #5561, .T. ) ;
#11756=ORIENTED_EDGE ( 'NONE', *, *, #24323, .T. ) ;
#11777=CARTESIAN_POINT ( 'NONE',  ( -0.01968503937007873988, -0.6102362204724409711, 0.000000000000000000 ) ) ;
#11793=VERTEX_POINT ( 'NONE', #5162 ) ;
#11814=EDGE_CURVE ( 'NONE', #14891, #23446, #16055, .T. ) ;
#11831=EDGE_CURVE ( 'NONE', #3892, #27393, #20776, .T. ) ;
#11861=DIRECTION ( 'NONE',  ( 0.000000000000000000, 0.000000000000000000, 1.000000000000000000 ) ) ;
#11903=SURFACE_STYLE_FILL_AREA ( #24891 ) ;
#11913=ORIENTED_EDGE ( 'NONE', *, *, #23131, .T. ) ;
#11915=ORIENTED_EDGE ( 'NONE', *, *, #3797, .T. ) ;
#11928=ORIENTED_EDGE ( 'NONE', *, *, #6645, .F. ) ;
#11975=MANIFOLD_SOLID_BREP ( 'Rear Bearing Cover', #22269 ) ;
#11985=SHAPE_REPRESENTATION_RELATIONSHIP ( 'NONE' , 'NONE' ,  #3575, #27550 ) ;
#11986=CYLINDRICAL_SURFACE ( 'NONE', #26879, 0.8267716535433071723 ) ;
#12001=VERTEX_POINT ( 'NONE', #27025 ) ;
#12010=DIRECTION ( 'NONE',  ( -1.000000000000000000, 0.000000000000000000, 0.000000000000000000 ) ) ;
#12043=VECTOR ( 'NONE', #13947, 39.37007874015748143 ) ;
#12065=CARTESIAN_POINT ( 'NONE',  ( -0.03937007874015747977, 0.5905511811023621549, 0.000000000000000000 ) ) ;
#12107=ORIENTED_EDGE ( 'NONE', *, *, #15288, .T. ) ;
#12147=AXIS2_PLACEMENT_3D ( 'NONE', #7460, #20746, #13972 ) ;
#12164=CARTESIAN_POINT ( 'NONE',  ( -0.2165354330708661457, 1.112204724409448842, 1.362057955744595713E-16 ) ) ;
#12173=( CONVERSION_BASED_UNIT ( 'INCH', #26723 ) LENGTH_UNIT ( ) NAMED_UNIT ( #16264 ) ) ;
#12221=VECTOR ( 'NONE', #16324, 39.37007874015748143 ) ;
#12248=EDGE_CURVE ( 'NONE', #27195, #14336, #26645, .T. ) ;
#12280=DIRECTION ( 'NONE',  ( 0.000000000000000000, 0.000000000000000000, 1.000000000000000000 ) ) ;
#12284=EDGE_CURVE ( 'NONE', #25761, #6278, #9957, .T. ) ;
#12332=ORIENTED_EDGE ( 'NONE', *, *, #19290, .T. ) ;
#12335=CARTESIAN_POINT ( 'NONE',  ( -0.5677492016568244093, -0.6030946203083737966, -0.9382345488188125193 ) ) ;
#12336=FACE_BOUND ( 'NONE', #22195, .T. ) ;
#12405=EDGE_CURVE ( 'NONE', #16795, #14218, #16041, .T. ) ;
#12415=AXIS2_PLACEMENT_3D ( 'NONE', #19850, #7001, #4589 ) ;
#12428=DIRECTION ( 'NONE',  ( 0.000000000000000000, 0.000000000000000000, 1.000000000000000000 ) ) ;
#12476=CARTESIAN_POINT ( 'NONE',  ( -0.5622644009080379757, -0.5390998427249246161, 0.9826767787474022242 ) ) ;
#12489=CARTESIAN_POINT ( 'NONE',  ( -0.3661417322834645272, 0.9448818897637796255, 0.1082677165354330451 ) ) ;
#12513=FACE_OUTER_BOUND ( 'NONE', #6390, .T. ) ;
#12542=ORIENTED_EDGE ( 'NONE', *, *, #7577, .T. ) ;
#12577=AXIS2_PLACEMENT_3D ( 'NONE', #21344, #1979, #10741 ) ;
#12587=CIRCLE ( 'NONE', #23892, 0.6889763779527560139 ) ;
#12595=CARTESIAN_POINT ( 'NONE',  ( -0.3661417322834645272, 0.9448818897637796255, -1.639108661417322569E-17 ) ) ;
#12619=CARTESIAN_POINT ( 'NONE',  ( -0.5776040203856925848, -0.4807978361611910945, 0.9954634121921446255 ) ) ;
#12656=DIRECTION ( 'NONE',  ( 1.000000000000000000, 0.000000000000000000, 0.000000000000000000 ) ) ;
#12658=CARTESIAN_POINT ( 'NONE',  ( -0.5511811023622047445, 0.000000000000000000, 0.000000000000000000 ) ) ;
#12659=CARTESIAN_POINT ( 'NONE',  ( -0.1968503937007874127, 0.9448818897637796255, -1.639108661417322569E-17 ) ) ;
#12684=DIRECTION ( 'NONE',  ( 1.000000000000000000, 0.000000000000000000, 0.000000000000000000 ) ) ;
#12685=VERTEX_POINT ( 'NONE', #6842 ) ;
#12692=EDGE_CURVE ( 'NONE', #11355, #9025, #19038, .T. ) ;
#12703=DIRECTION ( 'NONE',  ( 0.000000000000000000, -1.000000000000000000, 0.000000000000000000 ) ) ;
#12744=ORIENTED_EDGE ( 'NONE', *, *, #8516, .F. ) ;
#12776=FACE_OUTER_BOUND ( 'NONE', #27394, .T. ) ;
#12799=DIRECTION ( 'NONE',  ( 0.000000000000000000, 1.000000000000000000, 0.000000000000000000 ) ) ;
#12853=ORIENTED_EDGE ( 'NONE', *, *, #4650, .F. ) ;
#12857=EDGE_LOOP ( 'NONE', ( #2963, #3681 ) ) ;
#12872=LINE ( 'NONE', #15157, #2369 ) ;
#12899=CARTESIAN_POINT ( 'NONE',  ( -0.02559055118110236185, -0.8267716535433071723, 1.012503259137575512E-16 ) ) ;
#12913=DIRECTION ( 'NONE',  ( 0.000000000000000000, 1.000000000000000000, 0.000000000000000000 ) ) ;
#12920=DIRECTION ( 'NONE',  ( 0.000000000000000000, 1.000000000000000000, 0.000000000000000000 ) ) ;
#12932=CARTESIAN_POINT ( 'NONE',  ( -0.1771653543307086520, 0.7539370078740157410, 0.000000000000000000 ) ) ;
#12969=VERTEX_POINT ( 'NONE', #9300 ) ;
#12987=CIRCLE ( 'NONE', #10005, 1.092519685039370136 ) ;
#12989=CARTESIAN_POINT ( 'NONE',  ( -0.5700941239023215035, 1.111319899718911985, -0.06074667524653134393 ) ) ;
#12990=CARTESIAN_POINT ( 'NONE',  ( -0.4527559055118110520, 0.000000000000000000, 0.000000000000000000 ) ) ;
#13014=AXIS2_PLACEMENT_3D ( 'NONE', #16125, #15576, #24181 ) ;
#13023=VECTOR ( 'NONE', #15601, 39.37007874015748143 ) ;
#13076=DIRECTION ( 'NONE',  ( 0.000000000000000000, 1.000000000000000000, 0.000000000000000000 ) ) ;
#13081=VERTEX_POINT ( 'NONE', #12932 ) ;
#13089=ORIENTED_EDGE ( 'NONE', *, *, #17412, .F. ) ;
#13093=ORIENTED_EDGE ( 'NONE', *, *, #23388, .F. ) ;
#13101=DIRECTION ( 'NONE',  ( 1.000000000000000000, 0.000000000000000000, 0.000000000000000000 ) ) ;
#13146=DIRECTION ( 'NONE',  ( -1.000000000000000000, 0.000000000000000000, 0.000000000000000000 ) ) ;
#13158=DIRECTION ( 'NONE',  ( 0.000000000000000000, 1.000000000000000000, 0.000000000000000000 ) ) ;
#13177=CARTESIAN_POINT ( 'NONE',  ( -0.5905511811023621549, -1.092519685074702762, 0.000000000000000000 ) ) ;
#13202=AXIS2_PLACEMENT_3D ( 'NONE', #1579, #6253, #25597 ) ;
#13236=DIRECTION ( 'NONE',  ( 0.000000000000000000, -1.000000000000000000, 0.000000000000000000 ) ) ;
#13238=ORIENTED_EDGE ( 'NONE', *, *, #25655, .F. ) ;
#13253=CARTESIAN_POINT ( 'NONE',  ( -0.5664154050804837137, 1.115659691807800558, 0.04720470158372228747 ) ) ;
#13266=DIRECTION ( 'NONE',  ( -1.000000000000000000, 0.000000000000000000, 0.000000000000000000 ) ) ;
#13326=CARTESIAN_POINT ( 'NONE',  ( 2.664928230027803213, 0.9448818897637796255, 0.1082677165354330451 ) ) ;
#13331=DIRECTION ( 'NONE',  ( 0.7071067818211385081, -0.7071067805519564153, 0.000000000000000000 ) ) ;
#13332=ORIENTED_EDGE ( 'NONE', *, *, #11814, .F. ) ;
#13333=AXIS2_PLACEMENT_3D ( 'NONE', #20837, #2044, #1488 ) ;
#13386=AXIS2_PLACEMENT_3D ( 'NONE', #11016, #11289, #8755 ) ;
#13396=DIRECTION ( 'NONE',  ( -1.000000000000000000, 0.000000000000000000, 0.000000000000000000 ) ) ;
#13399=FACE_BOUND ( 'NONE', #80, .T. ) ;
#13440=CARTESIAN_POINT ( 'NONE',  ( -0.01968503937007873988, 0.6102362204724409711, -7.473238341253533632E-17 ) ) ;
#13467=DIRECTION ( 'NONE',  ( 1.000000000000000000, 0.000000000000000000, 0.000000000000000000 ) ) ;
#13472=CIRCLE ( 'NONE', #18447, 0.8267716535433071723 ) ;
#13480=ADVANCED_FACE ( 'NONE', ( #18799 ), #3728, .T. ) ;
#13487=DIRECTION ( 'NONE',  ( 0.000000000000000000, 0.000000000000000000, 1.000000000000000000 ) ) ;
#13517=ADVANCED_FACE ( 'NONE', ( #16702 ), #11390, .F. ) ;
#13518=CARTESIAN_POINT ( 'NONE',  ( -0.5610236220428271858, 1.122047244090071949, 1.311930826979132746E-15 ) ) ;
#13538=ORIENTED_EDGE ( 'NONE', *, *, #25590, .F. ) ;
#13543=EDGE_CURVE ( 'NONE', #25416, #27836, #12872, .T. ) ;
#13558=DIRECTION ( 'NONE',  ( 1.000000000000000000, 0.000000000000000000, 0.000000000000000000 ) ) ;
#13567=EDGE_LOOP ( 'NONE', ( #18956, #8570 ) ) ;
#13568=DIRECTION ( 'NONE',  ( -1.000000000000000000, 0.000000000000000000, 0.000000000000000000 ) ) ;
#13586=DIMENSIONAL_EXPONENTS ( 1.000000000000000000, 0.000000000000000000, 0.000000000000000000, 0.000000000000000000, 0.000000000000000000, 0.000000000000000000, 0.000000000000000000 ) ;
#13619=DIRECTION ( 'NONE',  ( 0.000000000000000000, 1.000000000000000000, 0.000000000000000000 ) ) ;
#13636=EDGE_CURVE ( 'NONE', #5917, #12685, #27681, .T. ) ;
#13639=DIRECTION ( 'NONE',  ( -0.7071067818211409506, -0.7071067805519539728, 0.000000000000000000 ) ) ;
#13670=DIRECTION ( 'NONE',  ( 0.000000000000000000, 0.000000000000000000, 1.000000000000000000 ) ) ;
#13688=DIRECTION ( 'NONE',  ( 0.000000000000000000, 1.000000000000000000, 0.000000000000000000 ) ) ;
#13772=VERTEX_POINT ( 'NONE', #5371 ) ;
#13786=ORIENTED_EDGE ( 'NONE', *, *, #21396, .F. ) ;
#13827=VERTEX_POINT ( 'NONE', #22458 ) ;
#13874=VECTOR ( 'NONE', #13331, 39.37007874015748854 ) ;
#13914=EDGE_CURVE ( 'NONE', #17036, #18321, #21805, .T. ) ;
#13931=CIRCLE ( 'NONE', #3080, 0.6995255587571318490 ) ;
#13947=DIRECTION ( 'NONE',  ( 1.000000000000000000, 0.000000000000000000, 0.000000000000000000 ) ) ;
#13972=DIRECTION ( 'NONE',  ( 0.000000000000000000, -1.000000000000000000, 0.000000000000000000 ) ) ;
#13994=DIRECTION ( 'NONE',  ( 0.000000000000000000, 0.000000000000000000, 1.000000000000000000 ) ) ;
#13996=AXIS2_PLACEMENT_3D ( 'NONE', #27606, #10204, #18821 ) ;
#14022=DIRECTION ( 'NONE',  ( 0.000000000000000000, 0.000000000000000000, 1.000000000000000000 ) ) ;
#14026=LINE ( 'NONE', #5111, #11686 ) ;
#14042=VERTEX_POINT ( 'NONE', #16669 ) ;
#14065=EDGE_LOOP ( 'NONE', ( #6851, #23109, #9751, #22203 ) ) ;
#14071=EDGE_CURVE ( 'NONE', #23853, #25692, #5929, .T. ) ;
#14100=ORIENTED_EDGE ( 'NONE', *, *, #8516, .T. ) ;
#14138=DIRECTION ( 'NONE',  ( -1.000000000000000000, 0.000000000000000000, 0.000000000000000000 ) ) ;
#14157=EDGE_CURVE ( 'NONE', #5023, #27816, #17304, .T. ) ;
#14176=EDGE_CURVE ( 'NONE', #3027, #3819, #20019, .T. ) ;
#14208=AXIS2_PLACEMENT_3D ( 'NONE', #24710, #14138, #13994 ) ;
#14218=VERTEX_POINT ( 'NONE', #5616 ) ;
#14258=DIRECTION ( 'NONE',  ( 1.000000000000000000, 0.000000000000000000, 0.000000000000000000 ) ) ;
#14273=B_SPLINE_CURVE_WITH_KNOTS ( 'NONE', 3,
 ( #8055, #16807, #16667, #1398 ),
 .UNSPECIFIED., .F., .F.,
 ( 4, 4 ),
 ( 0.000000000000000000, 0.08984410253495091203 ),
 .UNSPECIFIED. ) ;
#14278=CARTESIAN_POINT ( 'NONE',  ( -0.4783464566929133688, 0.9448818897637796255, -1.639108661417322569E-17 ) ) ;
#14296=AXIS2_PLACEMENT_3D ( 'NONE', #3278, #27038, #7685 ) ;
#14336=VERTEX_POINT ( 'NONE', #17880 ) ;
#14344=ORIENTED_EDGE ( 'NONE', *, *, #6448, .T. ) ;
#14384=AXIS2_PLACEMENT_3D ( 'NONE', #12990, #10874, #21896 ) ;
#14456=AXIS2_PLACEMENT_3D ( 'NONE', #11294, #15949, #7192 ) ;
#14473=CARTESIAN_POINT ( 'NONE',  ( -0.5640458768698323189, -0.5269038574489980364, 0.9872771499275302398 ) ) ;
#14479=CARTESIAN_POINT ( 'NONE',  ( -0.5751347059550788732, -0.6192722590600424626, -0.9188490092315169111 ) ) ;
#14507=AXIS2_PLACEMENT_3D ( 'NONE', #8573, #8841, #15224 ) ;
#14534=VERTEX_POINT ( 'NONE', #19958 ) ;
#14552=CARTESIAN_POINT ( 'NONE',  ( -0.1574803149606299191, 0.000000000000000000, 0.000000000000000000 ) ) ;
#14580=DIRECTION ( 'NONE',  ( 0.000000000000000000, 1.000000000000000000, 0.000000000000000000 ) ) ;
#14615=ORIENTED_EDGE ( 'NONE', *, *, #18002, .T. ) ;
#14624=DIRECTION ( 'NONE',  ( -1.000000000000000000, 0.000000000000000000, 0.000000000000000000 ) ) ;
#14653=CARTESIAN_POINT ( 'NONE',  ( -0.3937007874015748254, 0.000000000000000000, 0.000000000000000000 ) ) ;
#14666=DIRECTION ( 'NONE',  ( -1.000000000000000000, 0.000000000000000000, 0.000000000000000000 ) ) ;
#14672=DIRECTION ( 'NONE',  ( 1.000000000000000000, 0.000000000000000000, 0.000000000000000000 ) ) ;
#14705=AXIS2_PLACEMENT_3D ( 'NONE', #3905, #14672, #12799 ) ;
#14709=CYLINDRICAL_SURFACE ( 'NONE', #27541, 0.1771653543307086520 ) ;
#14750=EDGE_LOOP ( 'NONE', ( #4164, #3891, #26702, #8266 ) ) ;
#14764=ORIENTED_EDGE ( 'NONE', *, *, #11596, .F. ) ;
#14774=CARTESIAN_POINT ( 'NONE',  ( -0.5704976599510874768, -0.5016113632412458889, -0.9930866184833081478 ) ) ;
#14797=FACE_BOUND ( 'NONE', #20269, .T. ) ;
#14824=LINE ( 'NONE', #25536, #7996 ) ;
#14833=AXIS2_PLACEMENT_3D ( 'NONE', #989, #9576, #13688 ) ;
#14873=FACE_OUTER_BOUND ( 'NONE', #25962, .T. ) ;
#14891=VERTEX_POINT ( 'NONE', #2412 ) ;
#14902=CARTESIAN_POINT ( 'NONE',  ( -0.5811930530674194184, -0.4724394499398544278, -0.9954595798869386725 ) ) ;
#14924=EDGE_CURVE ( 'NONE', #26747, #22411, #6948, .T. ) ;
#14978=B_SPLINE_CURVE_WITH_KNOTS ( 'NONE', 3,
 ( #23375, #12619, #8386, #16565, #23226, #5850, #14473, #12476, #1596, #10200, #1738, #18818, #27455, #16716, #25475, #10349, #18965 ),
 .UNSPECIFIED., .F., .F.,
 ( 4, 2, 2, 1, 2, 2, 2, 2, 4 ),
 ( 0.08984410253495091203, 0.2036135897180814669, 0.2604983333096470011, 0.3173830769012125352, 0.4311525640843440477, 0.5449220512674757266, 0.6586915384506072391, 0.7724610256337387515, 1.000000000000000000 ),
 .UNSPECIFIED. ) ;
#14997=ORIENTED_EDGE ( 'NONE', *, *, #17288, .F. ) ;
#15009=ADVANCED_FACE ( 'NONE', ( #5806 ), #2954, .F. ) ;
#15040=AXIS2_PLACEMENT_3D ( 'NONE', #16429, #18246, #20806 ) ;
#15124=CARTESIAN_POINT ( 'NONE',  ( -0.5648342936079289167, 1.117528104686835722, 0.04027680511158680116 ) ) ;
#15132=CIRCLE ( 'NONE', #21871, 1.131889763779527547 ) ;
#15136=CARTESIAN_POINT ( 'NONE',  ( -0.5610237960480470853, 1.122047070076019448, -0.01921884795634628412 ) ) ;
#15157=CARTESIAN_POINT ( 'NONE',  ( -0.4783464566929133688, -0.4724409448818898127, -0.6411263657805729155 ) ) ;
#15160=ORIENTED_EDGE ( 'NONE', *, *, #7577, .F. ) ;
#15193=FACE_OUTER_BOUND ( 'NONE', #18897, .T. ) ;
#15207=AXIS2_PLACEMENT_3D ( 'NONE', #23309, #12684, #3936 ) ;
#15224=DIRECTION ( 'NONE',  ( 0.000000000000000000, 1.000000000000000000, 0.000000000000000000 ) ) ;
#15270=EDGE_CURVE ( 'NONE', #16472, #5917, #16913, .T. ) ;
#15275=CARTESIAN_POINT ( 'NONE',  ( -0.5636183736116697762, 1.118955382540468335, -0.03814816047951348488 ) ) ;
#15282=EDGE_LOOP ( 'NONE', ( #9454, #27413 ) ) ;
#15288=EDGE_CURVE ( 'NONE', #6278, #25761, #4705, .T. ) ;
#15297=DIRECTION ( 'NONE',  ( 0.000000000000000000, 1.000000000000000000, 0.000000000000000000 ) ) ;
#15338=AXIS2_PLACEMENT_3D ( 'NONE', #16543, #18946, #20934 ) ;
#15341=CONICAL_SURFACE ( 'NONE', #2656, 1.112204724409448842, 0.7853981624999977207 ) ;
#15356=AXIS2_PLACEMENT_3D ( 'NONE', #21808, #102, #2301 ) ;
#15359=CARTESIAN_POINT ( 'NONE',  ( 2.664928230027803213, -0.4724409448818898127, -0.8182917201112815953 ) ) ;
#15389=DIRECTION ( 'NONE',  ( 1.000000000000000000, 0.000000000000000000, 0.000000000000000000 ) ) ;
#15403=CARTESIAN_POINT ( 'NONE',  ( -0.5675505653814777451, 1.114319256831761251, 0.05180297602549875646 ) ) ;
#15412=FACE_OUTER_BOUND ( 'NONE', #7327, .T. ) ;
#15420=CYLINDRICAL_SURFACE ( 'NONE', #14384, 0.6889763779527560139 ) ;
#15426=CARTESIAN_POINT ( 'NONE',  ( -0.3661417322834645272, -0.4724409448818898127, 0.9954570744419902750 ) ) ;
#15468=DIRECTION ( 'NONE',  ( -1.000000000000000000, 0.000000000000000000, 0.000000000000000000 ) ) ;
#15476=LINE ( 'NONE', #4712, #6433 ) ;
#15497=ORIENTED_EDGE ( 'NONE', *, *, #3325, .T. ) ;
#15510=FACE_OUTER_BOUND ( 'NONE', #7650, .T. ) ;
#15530=AXIS2_PLACEMENT_3D ( 'NONE', #10023, #3809, #12428 ) ;
#15565=DIRECTION ( 'NONE',  ( -1.000000000000000000, 0.000000000000000000, 0.000000000000000000 ) ) ;
#15576=DIRECTION ( 'NONE',  ( 1.000000000000000000, 0.000000000000000000, 0.000000000000000000 ) ) ;
#15601=DIRECTION ( 'NONE',  ( -1.000000000000000000, 0.000000000000000000, 0.000000000000000000 ) ) ;
#15641=DIRECTION ( 'NONE',  ( -1.000000000000000000, 0.000000000000000000, 0.000000000000000000 ) ) ;
#15707=EDGE_LOOP ( 'NONE', ( #27548, #1091 ) ) ;
#15762=ADVANCED_FACE ( 'NONE', ( #9521 ), #20314, .F. ) ;
#15786=AXIS2_PLACEMENT_3D ( 'NONE', #6144, #8247, #25759 ) ;
#15801=DIRECTION ( 'NONE',  ( 0.000000000000000000, -1.000000000000000000, 0.000000000000000000 ) ) ;
#15804=CONICAL_SURFACE ( 'NONE', #7223, 1.112204724409448842, 0.7853981624999977207 ) ;
#15870=DIRECTION ( 'NONE',  ( -1.000000000000000000, 0.000000000000000000, 0.000000000000000000 ) ) ;
#15891=ORIENTED_EDGE ( 'NONE', *, *, #20124, .F. ) ;
#15935=DIRECTION ( 'NONE',  ( -1.000000000000000000, 0.000000000000000000, 0.000000000000000000 ) ) ;
#15939=ORIENTED_EDGE ( 'NONE', *, *, #24237, .F. ) ;
#15949=DIRECTION ( 'NONE',  ( -1.000000000000000000, 0.000000000000000000, 0.000000000000000000 ) ) ;
#16005=( NAMED_UNIT ( * ) PLANE_ANGLE_UNIT ( ) SI_UNIT ( $, .RADIAN. ) ) ;
#16014=DIRECTION ( 'NONE',  ( -1.000000000000000000, 0.000000000000000000, 0.000000000000000000 ) ) ;
#16041=LINE ( 'NONE', #648, #12221 ) ;
#16055=LINE ( 'NONE', #18135, #23947 ) ;
#16056=AXIS2_PLACEMENT_3D ( 'NONE', #26421, #20356, #20208 ) ;
#16095=VERTEX_POINT ( 'NONE', #5992 ) ;
#16111=EDGE_CURVE ( 'NONE', #5538, #16472, #14978, .T. ) ;
#16112=FACE_OUTER_BOUND ( 'NONE', #23545, .T. ) ;
#16125=CARTESIAN_POINT ( 'NONE',  ( -0.1870078740157480324, 0.000000000000000000, 0.000000000000000000 ) ) ;
#16129=DIRECTION ( 'NONE',  ( 1.000000000000000000, 0.000000000000000000, 0.000000000000000000 ) ) ;
#16132=DIRECTION ( 'NONE',  ( 0.000000000000000000, 0.000000000000000000, 1.000000000000000000 ) ) ;
#16187=B_SPLINE_CURVE_WITH_KNOTS ( 'NONE', 3,
 ( #8297, #25525, #25663, #6317 ),
 .UNSPECIFIED., .F., .F.,
 ( 4, 4 ),
 ( 0.9101643785100869133, 1.000000000000000000 ),
 .UNSPECIFIED. ) ;
#16205=EDGE_CURVE ( 'NONE', #22689, #14042, #22813, .T. ) ;
#16219=VERTEX_POINT ( 'NONE', #24184 ) ;
#16247=ORIENTED_EDGE ( 'NONE', *, *, #17918, .F. ) ;
#16253=CARTESIAN_POINT ( 'NONE',  ( 2.664928230027803213, -0.4724409448818898127, 0.8182917201112815953 ) ) ;
#16264=DIMENSIONAL_EXPONENTS ( 1.000000000000000000, 0.000000000000000000, 0.000000000000000000, 0.000000000000000000, 0.000000000000000000, 0.000000000000000000, 0.000000000000000000 ) ;
#16304=LINE ( 'NONE', #26889, #9625 ) ;
#16310=DIRECTION ( 'NONE',  ( 1.000000000000000000, 0.000000000000000000, 0.000000000000000000 ) ) ;
#16313=ORIENTED_EDGE ( 'NONE', *, *, #13914, .F. ) ;
#16324=DIRECTION ( 'NONE',  ( -0.9659258263664933786, 0.2588190448135666011, 3.169619147893097007E-17 ) ) ;
#16336=DIRECTION ( 'NONE',  ( -1.000000000000000000, 0.000000000000000000, 0.000000000000000000 ) ) ;
#16344=CARTESIAN_POINT ( 'NONE',  ( -0.1968503937007874127, -0.4724409448818898127, -0.7100240035758484947 ) ) ;
#16361=ADVANCED_FACE ( 'NONE', ( #18355 ), #9606, .T. ) ;
#16376=CIRCLE ( 'NONE', #18583, 1.092519685039370136 ) ;
#16429=CARTESIAN_POINT ( 'NONE',  ( -0.5511811023622047445, 0.000000000000000000, 0.000000000000000000 ) ) ;
#16472=VERTEX_POINT ( 'NONE', #3973 ) ;
#16543=CARTESIAN_POINT ( 'NONE',  ( -0.3661417322834645272, -0.4724409448818898127, -0.8182917201112815953 ) ) ;
#16565=CARTESIAN_POINT ( 'NONE',  ( -0.5704973819974966665, -0.5016125552370697127, 0.9930863283245008333 ) ) ;
#16568=CARTESIAN_POINT ( 'NONE',  ( -0.3661417322834645272, -0.4724409448818898127, 0.8182917201112815953 ) ) ;
#16590=ORIENTED_EDGE ( 'NONE', *, *, #20313, .T. ) ;
#16601=PLANE ( 'NONE',  #13333 ) ;
#16613=VECTOR ( 'NONE', #7196, 39.37007874015748143 ) ;
#16654=AXIS2_PLACEMENT_3D ( 'NONE', #6717, #13467, #12920 ) ;
#16667=CARTESIAN_POINT ( 'NONE',  ( -0.5840204509605140260, -0.4658379333985104287, 0.9954608945792949859 ) ) ;
#16669=CARTESIAN_POINT ( 'NONE',  ( -0.5905511811023621549, 1.087444635826771533, -0.1051828227901525498 ) ) ;
#16698=ORIENTED_EDGE ( 'NONE', *, *, #27300, .F. ) ;
#16702=FACE_OUTER_BOUND ( 'NONE', #9489, .T. ) ;
#16716=CARTESIAN_POINT ( 'NONE',  ( -0.5677494271516411173, -0.6030950601078316486, 0.9382339938615534836 ) ) ;
#16730=AXIS2_PLACEMENT_3D ( 'NONE', #7864, #1234, #3463 ) ;
#16741=ADVANCED_FACE ( 'NONE', ( #26264, #1496 ), #7060, .T. ) ;
#16744=FACE_BOUND ( 'NONE', #6163, .T. ) ;
#16753=EDGE_CURVE ( 'NONE', #22409, #25416, #26168, .T. ) ;
#16768=LINE ( 'NONE', #18441, #21163 ) ;
#16769=ORIENTED_EDGE ( 'NONE', *, *, #9735, .T. ) ;
#16777=CARTESIAN_POINT ( 'NONE',  ( -0.05118110236220472370, -0.8267716535433071723, 1.012503259137575512E-16 ) ) ;
#16779=ORIENTED_EDGE ( 'NONE', *, *, #2760, .T. ) ;
#16795=VERTEX_POINT ( 'NONE', #7471 ) ;
#16807=CARTESIAN_POINT ( 'NONE',  ( -0.5871411068728082938, -0.4592309206872642879, 0.9950886776261244071 ) ) ;
#16814=DIRECTION ( 'NONE',  ( 0.000000000000000000, -1.000000000000000000, 0.000000000000000000 ) ) ;
#16822=ORIENTED_EDGE ( 'NONE', *, *, #27734, .F. ) ;
#16827=ORIENTED_EDGE ( 'NONE', *, *, #11608, .T. ) ;
#16828=CARTESIAN_POINT ( 'NONE',  ( -0.5858067486093416765, 1.092930385925676040, -0.09774754414358965970 ) ) ;
#16846=AXIS2_PLACEMENT_3D ( 'NONE', #21215, #1855, #19080 ) ;
#16871=CARTESIAN_POINT ( 'NONE',  ( -0.5660396215081976434, -0.5184600247624503444, -0.9894322414029975699 ) ) ;
#16913=CIRCLE ( 'NONE', #4285, 1.092519685039370136 ) ;
#16936=ORIENTED_EDGE ( 'NONE', *, *, #14157, .T. ) ;
#16999=DIRECTION ( 'NONE',  ( 0.000000000000000000, -1.000000000000000000, 0.000000000000000000 ) ) ;
#17009=CARTESIAN_POINT ( 'NONE',  ( -0.5905511811023621549, 0.9448818897637796255, -1.639108661417322569E-17 ) ) ;
#17017=EDGE_CURVE ( 'NONE', #25537, #18462, #3146, .T. ) ;
#17018=PRODUCT_DEFINITION_CONTEXT ( 'detailed design', #4568, 'design' ) ;
#17027=EDGE_CURVE ( 'NONE', #25537, #3239, #23477, .T. ) ;
#17036=VERTEX_POINT ( 'NONE', #4012 ) ;
#17077=FACE_OUTER_BOUND ( 'NONE', #6193, .T. ) ;
#17127=EDGE_LOOP ( 'NONE', ( #8582, #25260, #12332, #22773 ) ) ;
#17159=DIRECTION ( 'NONE',  ( 0.000000000000000000, 0.000000000000000000, 1.000000000000000000 ) ) ;
#17203=ADVANCED_FACE ( 'NONE', ( #12336, #1600 ), #23231, .T. ) ;
#17222=CARTESIAN_POINT ( 'NONE',  ( -0.05118110236220472370, 0.000000000000000000, 0.000000000000000000 ) ) ;
#17284=LINE ( 'NONE', #13440, #24951 ) ;
#17288=EDGE_CURVE ( 'NONE', #23446, #12969, #470, .T. ) ;
#17304=CIRCLE ( 'NONE', #21388, 0.8267716535433071723 ) ;
#17412=EDGE_CURVE ( 'NONE', #18929, #8838, #22436, .T. ) ;
#17449=DIRECTION ( 'NONE',  ( 0.000000000000000000, 0.000000000000000000, 1.000000000000000000 ) ) ;
#17455=CARTESIAN_POINT ( 'NONE',  ( -0.1771653543307086520, 0.000000000000000000, 0.000000000000000000 ) ) ;
#17488=EDGE_LOOP ( 'NONE', ( #26933, #10089, #17719, #19187 ) ) ;
#17494=CARTESIAN_POINT ( 'NONE',  ( -0.5636180690721820374, 1.118968434182232574, 0.03326447829218234092 ) ) ;
#17513=ORIENTED_EDGE ( 'NONE', *, *, #12405, .F. ) ;
#17532=CARTESIAN_POINT ( 'NONE',  ( -0.5905511811023621549, 0.000000000000000000, 0.000000000000000000 ) ) ;
#17552=ORIENTED_EDGE ( 'NONE', *, *, #4591, .F. ) ;
#17553=ORIENTED_EDGE ( 'NONE', *, *, #5688, .T. ) ;
#17555=CONICAL_SURFACE ( 'NONE', #24299, 1.112204724409448842, 0.7853981625000011624 ) ;
#17562=ORIENTED_EDGE ( 'NONE', *, *, #23316, .F. ) ;
#17602=VERTEX_POINT ( 'NONE', #15426 ) ;
#17604=ORIENTED_EDGE ( 'NONE', *, *, #24323, .F. ) ;
#17611=ORIENTED_EDGE ( 'NONE', *, *, #25900, .F. ) ;
#17619=ORIENTED_EDGE ( 'NONE', *, *, #11814, .T. ) ;
#17636=PLANE ( 'NONE',  #18932 ) ;
#17641=FACE_OUTER_BOUND ( 'NONE', #6758, .T. ) ;
#17676=CARTESIAN_POINT ( 'NONE',  ( -0.3149606299212598381, 0.000000000000000000, 0.000000000000000000 ) ) ;
#17705=EDGE_LOOP ( 'NONE', ( #22716, #10947, #19048, #8779 ) ) ;
#17707=LINE ( 'NONE', #26331, #25664 ) ;
#17718=APPLICATION_CONTEXT ( 'automotive_design' ) ;
#17719=ORIENTED_EDGE ( 'NONE', *, *, #17744, .T. ) ;
#17744=EDGE_CURVE ( 'NONE', #22551, #13827, #7336, .T. ) ;
#17760=CARTESIAN_POINT ( 'NONE',  ( -0.5905511811023621549, -0.4724409448818898127, -0.8182917201112815953 ) ) ;
#17780=EDGE_CURVE ( 'NONE', #12969, #23446, #4441, .T. ) ;
#17790=DIRECTION ( 'NONE',  ( 0.000000000000000000, -1.000000000000000000, 0.000000000000000000 ) ) ;
#17880=CARTESIAN_POINT ( 'NONE',  ( -0.1968503937007874127, 0.9448818897637796255, -0.1082677165354330867 ) ) ;
#17904=DIRECTION ( 'NONE',  ( -1.000000000000000000, 0.000000000000000000, 0.000000000000000000 ) ) ;
#17918=EDGE_CURVE ( 'NONE', #10221, #1935, #20215, .T. ) ;
#17921=EDGE_CURVE ( 'NONE', #3819, #3027, #22478, .T. ) ;
#17930=DIRECTION ( 'NONE',  ( -1.000000000000000000, 0.000000000000000000, 0.000000000000000000 ) ) ;
#17988=CIRCLE ( 'NONE', #15356, 0.1771653543307086798 ) ;
#18002=EDGE_CURVE ( 'NONE', #21048, #3293, #22954, .T. ) ;
#18004=CARTESIAN_POINT ( 'NONE',  ( -0.01968503937007873988, 0.000000000000000000, 0.000000000000000000 ) ) ;
#18052=DIRECTION ( 'NONE',  ( -1.000000000000000000, 0.000000000000000000, 0.000000000000000000 ) ) ;
#18066=VECTOR ( 'NONE', #4878, 39.37007874015748854 ) ;
#18072=ADVANCED_FACE ( 'NONE', ( #7436 ), #23417, .F. ) ;
#18135=CARTESIAN_POINT ( 'NONE',  ( -0.4527559055118110520, -0.6889763779527560139, 8.437527159479796553E-17 ) ) ;
#18193=CARTESIAN_POINT ( 'NONE',  ( -0.1968503937007874127, -0.4724409448818898127, -0.8182917201112815953 ) ) ;
#18207=DIRECTION ( 'NONE',  ( 0.000000000000000000, 1.000000000000000000, 0.000000000000000000 ) ) ;
#18228=CARTESIAN_POINT ( 'NONE',  ( -0.1141732283464566844, -0.7539370078740157410, 9.233065434516462138E-17 ) ) ;
#18246=DIRECTION ( 'NONE',  ( 1.000000000000000000, 0.000000000000000000, 0.000000000000000000 ) ) ;
#18273=AXIS2_PLACEMENT_3D ( 'NONE', #10375, #23674, #3887 ) ;
#18291=AXIS2_PLACEMENT_3D ( 'NONE', #18193, #15565, #24227 ) ;
#18305=CARTESIAN_POINT ( 'NONE',  ( -0.5811915241081616612, -0.4724399524670138684, 0.9954595399565421276 ) ) ;
#18321=VERTEX_POINT ( 'NONE', #11466 ) ;
#18352=LINE ( 'NONE', #9462, #26106 ) ;
#18355=FACE_OUTER_BOUND ( 'NONE', #14065, .T. ) ;
#18361=ORIENTED_EDGE ( 'NONE', *, *, #24424, .T. ) ;
#18367=LINE ( 'NONE', #18228, #18862 ) ;
#18372=( LENGTH_UNIT ( ) NAMED_UNIT ( * ) SI_UNIT ( $, .METRE. ) ) ;
#18394=CARTESIAN_POINT ( 'NONE',  ( -0.1870078740157480324, 0.000000000000000000, 0.000000000000000000 ) ) ;
#18441=CARTESIAN_POINT ( 'NONE',  ( -0.4527559055118110520, 0.6889763779527560139, 0.000000000000000000 ) ) ;
#18445=DIRECTION ( 'NONE',  ( 0.000000000000000000, 0.000000000000000000, 1.000000000000000000 ) ) ;
#18447=AXIS2_PLACEMENT_3D ( 'NONE', #6800, #69, #15297 ) ;
#18457=ORIENTED_EDGE ( 'NONE', *, *, #16753, .F. ) ;
#18459=DIRECTION ( 'NONE',  ( 0.000000000000000000, 1.000000000000000000, 0.000000000000000000 ) ) ;
#18462=VERTEX_POINT ( 'NONE', #4051 ) ;
#18470=EDGE_CURVE ( 'NONE', #16095, #14891, #12587, .T. ) ;
#18505=DIRECTION ( 'NONE',  ( -0.9659258263664933786, 0.2588190448135661570, 3.169619147893090844E-17 ) ) ;
#18532=ORIENTED_EDGE ( 'NONE', *, *, #17744, .F. ) ;
#18537=CYLINDRICAL_SURFACE ( 'NONE', #1980, 0.1082677165354330312 ) ;
#18578=AXIS2_PLACEMENT_3D ( 'NONE', #22986, #14666, #10242 ) ;
#18583=AXIS2_PLACEMENT_3D ( 'NONE', #20947, #14624, #16999 ) ;
#18601=CARTESIAN_POINT ( 'NONE',  ( -0.5905511811023621549, -0.4526313213353566622, -0.9943460912301791410 ) ) ;
#18628=VECTOR ( 'NONE', #13101, 39.37007874015748143 ) ;
#18643=CARTESIAN_POINT ( 'NONE',  ( -0.5905511811023621549, 0.000000000000000000, 0.000000000000000000 ) ) ;
#18646=CARTESIAN_POINT ( 'NONE',  ( -0.1968503937007874127, -0.4724409448818898127, -0.9265594366467145848 ) ) ;
#18653=ADVANCED_FACE ( 'NONE', ( #25118 ), #1767, .F. ) ;
#18670=ORIENTED_EDGE ( 'NONE', *, *, #16205, .F. ) ;
#18726=CIRCLE ( 'NONE', #21457, 0.1771653543307086520 ) ;
#18729=DIRECTION ( 'NONE',  ( -1.000000000000000000, 0.000000000000000000, 0.000000000000000000 ) ) ;
#18736=ORIENTED_EDGE ( 'NONE', *, *, #11218, .F. ) ;
#18746=ORIENTED_EDGE ( 'NONE', *, *, #15288, .F. ) ;
#18799=FACE_OUTER_BOUND ( 'NONE', #24922, .T. ) ;
#18818=CARTESIAN_POINT ( 'NONE',  ( -0.5626607827700350617, -0.5839868939222687683, 0.9562171551394879065 ) ) ;
#18821=DIRECTION ( 'NONE',  ( 0.000000000000000000, 0.000000000000000000, 1.000000000000000000 ) ) ;
#18852=CARTESIAN_POINT ( 'NONE',  ( -0.4783464566929133688, 0.9448818897637796255, -0.1771653543307086520 ) ) ;
#18859=FACE_OUTER_BOUND ( 'NONE', #2758, .T. ) ;
#18862=VECTOR ( 'NONE', #11475, 39.37007874015748143 ) ;
#18869=EDGE_CURVE ( 'NONE', #1935, #10221, #26023, .T. ) ;
#18897=EDGE_LOOP ( 'NONE', ( #23723, #1121 ) ) ;
#18910=CYLINDRICAL_SURFACE ( 'NONE', #27706, 0.1771653543307086520 ) ;
#18925=CARTESIAN_POINT ( 'NONE',  ( -0.03937007874015747977, -0.8267716535433071723, 1.012503259137575512E-16 ) ) ;
#18929=VERTEX_POINT ( 'NONE', #16344 ) ;
#18932=AXIS2_PLACEMENT_3D ( 'NONE', #2523, #13396, #19483 ) ;
#18946=DIRECTION ( 'NONE',  ( -1.000000000000000000, 0.000000000000000000, 0.000000000000000000 ) ) ;
#18956=ORIENTED_EDGE ( 'NONE', *, *, #25516, .F. ) ;
#18965=CARTESIAN_POINT ( 'NONE',  ( -0.5905511811023621549, -0.6348133144914153148, 0.8891632684400255782 ) ) ;
#18985=AXIS2_PLACEMENT_3D ( 'NONE', #15359, #1918, #17449 ) ;
#18992=ORIENTED_EDGE ( 'NONE', *, *, #10679, .T. ) ;
#19008=CARTESIAN_POINT ( 'NONE',  ( -0.2362204724409449064, 0.000000000000000000, 0.000000000000000000 ) ) ;
#19029=VERTEX_POINT ( 'NONE', #9039 ) ;
#19038=CIRCLE ( 'NONE', #5035, 0.1082677165354330312 ) ;
#19048=ORIENTED_EDGE ( 'NONE', *, *, #17017, .T. ) ;
#19050=AXIS2_PLACEMENT_3D ( 'NONE', #2380, #24271, #15801 ) ;
#19080=DIRECTION ( 'NONE',  ( 0.000000000000000000, 0.000000000000000000, 1.000000000000000000 ) ) ;
#19118=AXIS2_PLACEMENT_3D ( 'NONE', #18394, #7539, #24906 ) ;
#19123=ADVANCED_FACE ( 'NONE', ( #13399, #17641 ), #23884, .T. ) ;
#19153=DIRECTION ( 'NONE',  ( 1.000000000000000000, 0.000000000000000000, 0.000000000000000000 ) ) ;
#19187=ORIENTED_EDGE ( 'NONE', *, *, #26709, .F. ) ;
#19203=DIRECTION ( 'NONE',  ( 1.000000000000000000, 0.000000000000000000, 0.000000000000000000 ) ) ;
#19208=ORIENTED_EDGE ( 'NONE', *, *, #6448, .F. ) ;
#19209=FACE_BOUND ( 'NONE', #7424, .T. ) ;
#19254=DIRECTION ( 'NONE',  ( 0.7071067818211370648, -0.7071067805519580807, 0.000000000000000000 ) ) ;
#19268=CARTESIAN_POINT ( 'NONE',  ( -2.185478346456693112E-16, 0.6299212598071869396, -7.714310545377398371E-17 ) ) ;
#19278=( GEOMETRIC_REPRESENTATION_CONTEXT ( 3 ) GLOBAL_UNCERTAINTY_ASSIGNED_CONTEXT ( ( #27126 ) ) GLOBAL_UNIT_ASSIGNED_CONTEXT ( ( #27106, #5493, #22870 ) ) REPRESENTATION_CONTEXT ( 'NONE', 'WORKASPACE' ) ) ;
#19290=EDGE_CURVE ( 'NONE', #5023, #14218, #4293, .T. ) ;
#19324=ORIENTED_EDGE ( 'NONE', *, *, #12248, .T. ) ;
#19333=ORIENTED_EDGE ( 'NONE', *, *, #7653, .F. ) ;
#19338=EDGE_CURVE ( 'NONE', #8838, #18929, #11100, .T. ) ;
#19342=AXIS2_PLACEMENT_3D ( 'NONE', #16253, #12010, #11861 ) ;
#19353=ORIENTED_EDGE ( 'NONE', *, *, #20623, .F. ) ;
#19354=CARTESIAN_POINT ( 'NONE',  ( -0.5816225468157798506, 1.097802432538817152, -0.08994119036359567165 ) ) ;
#19358=ORIENTED_EDGE ( 'NONE', *, *, #27124, .T. ) ;
#19371=CARTESIAN_POINT ( 'NONE',  ( -0.5905511811023621549, -0.4724409448818898127, -0.8182917201112815953 ) ) ;
#19372=CIRCLE ( 'NONE', #22060, 0.1082677165354330312 ) ;
#19382=AXIS2_PLACEMENT_3D ( 'NONE', #12659, #27511, #8154 ) ;
#19383=ORIENTED_EDGE ( 'NONE', *, *, #26481, .T. ) ;
#19407=ADVANCED_FACE ( 'NONE', ( #27291 ), #11986, .T. ) ;
#19448=LINE ( 'NONE', #2079, #18066 ) ;
#19449=ORIENTED_EDGE ( 'NONE', *, *, #13543, .T. ) ;
#19483=DIRECTION ( 'NONE',  ( 0.000000000000000000, 0.000000000000000000, 1.000000000000000000 ) ) ;
#19485=LINE ( 'NONE', #7049, #2382 ) ;
#19488=CARTESIAN_POINT ( 'NONE',  ( -0.5694559772926249819, 1.112071903501507641, -0.05864771439935212438 ) ) ;
#19525=ADVANCED_FACE ( 'NONE', ( #8135, #16744, #14797, #1625, #25505 ), #16601, .T. ) ;
#19563=CARTESIAN_POINT ( 'NONE',  ( -0.4783464566929133688, -0.4724409448818898127, 0.8182917201112815953 ) ) ;
#19659=VECTOR ( 'NONE', #18505, 39.37007874015748854 ) ;
#19687=ORIENTED_EDGE ( 'NONE', *, *, #12692, .T. ) ;
#19723=CIRCLE ( 'NONE', #1676, 0.1771653543307086520 ) ;
#19739=CARTESIAN_POINT ( 'NONE',  ( -0.3937007874015748254, -1.131889763779527547, 1.386165176200252194E-16 ) ) ;
#19810=DIRECTION ( 'NONE',  ( 0.7071067818211370648, 0.7071067805519580807, -8.659560554583453627E-17 ) ) ;
#19850=CARTESIAN_POINT ( 'NONE',  ( -0.5708661417322835607, 0.000000000000000000, 0.000000000000000000 ) ) ;
#19936=DIRECTION ( 'NONE',  ( 1.000000000000000000, 0.000000000000000000, 0.000000000000000000 ) ) ;
#19958=CARTESIAN_POINT ( 'NONE',  ( -0.5905511811023621549, -0.4526313213353574949, 0.9943460912301771426 ) ) ;
#19979=AXIS2_PLACEMENT_3D ( 'NONE', #17532, #13558, #17790 ) ;
#20019=CIRCLE ( 'NONE', #23638, 0.1082677165354330728 ) ;
#20026=CARTESIAN_POINT ( 'NONE',  ( -0.5905511811023621549, -0.6995255587508188988, 0.000000000000000000 ) ) ;
#20033=CARTESIAN_POINT ( 'NONE',  ( -0.3149606299212598381, -0.5905511811023621549, 7.232166136696967594E-17 ) ) ;
#20039=ORIENTED_EDGE ( 'NONE', *, *, #26820, .F. ) ;
#20056=DIRECTION ( 'NONE',  ( -1.000000000000000000, 0.000000000000000000, 0.000000000000000000 ) ) ;
#20069=ORIENTED_EDGE ( 'NONE', *, *, #11730, .F. ) ;
#20124=EDGE_CURVE ( 'NONE', #6094, #13081, #10191, .T. ) ;
#20155=CARTESIAN_POINT ( 'NONE',  ( -0.5610236220428271858, 1.122047244090071949, 1.311930826979132746E-15 ) ) ;
#20165=EDGE_LOOP ( 'NONE', ( #19383, #2643, #20211, #18532 ) ) ;
#20198=CYLINDRICAL_SURFACE ( 'NONE', #19342, 0.1082677165354330312 ) ;
#20208=DIRECTION ( 'NONE',  ( 0.000000000000000000, 1.000000000000000000, 0.000000000000000000 ) ) ;
#20211=ORIENTED_EDGE ( 'NONE', *, *, #20729, .F. ) ;
#20215=CIRCLE ( 'NONE', #2605, 0.5905511811023621549 ) ;
#20216=ORIENTED_EDGE ( 'NONE', *, *, #17921, .T. ) ;
#20250=CARTESIAN_POINT ( 'NONE',  ( -0.1968503937007874127, -0.4724409448818898127, 0.9265594366467145848 ) ) ;
#20269=EDGE_LOOP ( 'NONE', ( #19324, #14344 ) ) ;
#20298=AXIS2_PLACEMENT_3D ( 'NONE', #22167, #7329, #6929 ) ;
#20313=EDGE_CURVE ( 'NONE', #3232, #5851, #18352, .T. ) ;
#20314=CYLINDRICAL_SURFACE ( 'NONE', #25517, 0.5905511811023621549 ) ;
#20329=FACE_OUTER_BOUND ( 'NONE', #11337, .T. ) ;
#20336=CARTESIAN_POINT ( 'NONE',  ( -0.05118110236220472370, -0.7539370078740157410, 9.233065434516462138E-17 ) ) ;
#20346=DIRECTION ( 'NONE',  ( 1.000000000000000000, 0.000000000000000000, 0.000000000000000000 ) ) ;
#20356=DIRECTION ( 'NONE',  ( 1.000000000000000000, 0.000000000000000000, 0.000000000000000000 ) ) ;
#20380=ADVANCED_FACE ( 'NONE', ( #7498 ), #26423, .T. ) ;
#20398=ORIENTED_EDGE ( 'NONE', *, *, #20995, .T. ) ;
#20404=ORIENTED_EDGE ( 'NONE', *, *, #20729, .T. ) ;
#20424=ORIENTED_EDGE ( 'NONE', *, *, #18869, .F. ) ;
#20483=DIRECTION ( 'NONE',  ( 0.000000000000000000, 1.000000000000000000, 0.000000000000000000 ) ) ;
#20516=FACE_OUTER_BOUND ( 'NONE', #7246, .T. ) ;
#20560=AXIS2_PLACEMENT_3D ( 'NONE', #14653, #25353, #12913 ) ;
#20579=AXIS2_PLACEMENT_3D ( 'NONE', #26026, #2423, #13158 ) ;
#20623=EDGE_CURVE ( 'NONE', #13081, #6278, #23615, .T. ) ;
#20634=ADVANCED_FACE ( 'NONE', ( #27705 ), #15420, .F. ) ;
#20638=ORIENTED_EDGE ( 'NONE', *, *, #26548, .T. ) ;
#20646=CARTESIAN_POINT ( 'NONE',  ( -0.5708661417322835607, 0.6942509683549429322, 8.502122262008311951E-17 ) ) ;
#20674=CARTESIAN_POINT ( 'NONE',  ( -0.4783464566929133688, -0.4724409448818898127, 0.9954570744419902750 ) ) ;
#20691=ADVANCED_FACE ( 'NONE', ( #14873 ), #17555, .T. ) ;
#20697=ADVANCED_FACE ( 'NONE', ( #315 ), #25720, .F. ) ;
#20729=EDGE_CURVE ( 'NONE', #13827, #8922, #25206, .T. ) ;
#20746=DIRECTION ( 'NONE',  ( 1.000000000000000000, 0.000000000000000000, 0.000000000000000000 ) ) ;
#20776=CIRCLE ( 'NONE', #7698, 0.1082677165354330312 ) ;
#20777=DIRECTION ( 'NONE',  ( 1.000000000000000000, 0.000000000000000000, 0.000000000000000000 ) ) ;
#20789=DIRECTION ( 'NONE',  ( -0.7071067818211409506, 0.7071067805519539728, 8.659560554583403090E-17 ) ) ;
#20806=DIRECTION ( 'NONE',  ( 0.000000000000000000, -1.000000000000000000, 0.000000000000000000 ) ) ;
#20837=CARTESIAN_POINT ( 'NONE',  ( -0.1968503937007874127, 0.9793307086614173596, 0.000000000000000000 ) ) ;
#20858=CIRCLE ( 'NONE', #18578, 1.131889763779527547 ) ;
#20860=ADVANCED_FACE ( 'NONE', ( #23264, #12513 ), #1771, .T. ) ;
#20865=CONICAL_SURFACE ( 'NONE', #3697, 0.6942509683549429322, 0.2617993875000015902 ) ;
#20892=FACE_OUTER_BOUND ( 'NONE', #2103, .T. ) ;
#20906=CARTESIAN_POINT ( 'NONE',  ( -0.5905511811023621549, 0.000000000000000000, 0.000000000000000000 ) ) ;
#20914=ORIENTED_EDGE ( 'NONE', *, *, #13636, .T. ) ;
#20927=EDGE_CURVE ( 'NONE', #10221, #3239, #17707, .T. ) ;
#20934=DIRECTION ( 'NONE',  ( 0.000000000000000000, 0.000000000000000000, 1.000000000000000000 ) ) ;
#20947=CARTESIAN_POINT ( 'NONE',  ( -0.1968503937007874127, 0.000000000000000000, 0.000000000000000000 ) ) ;
#20954=CARTESIAN_POINT ( 'NONE',  ( -0.5609635780474857558, -0.5548708040265607488, -0.9753554781212179225 ) ) ;
#20995=EDGE_CURVE ( 'NONE', #17602, #5538, #11495, .T. ) ;
#21038=DIRECTION ( 'NONE',  ( -1.000000000000000000, 0.000000000000000000, 0.000000000000000000 ) ) ;
#21048=VERTEX_POINT ( 'NONE', #20250 ) ;
#21069=ADVANCED_FACE ( 'NONE', ( #26740 ), #22515, .T. ) ;
#21095=DIRECTION ( 'NONE',  ( 0.000000000000000000, 0.000000000000000000, 1.000000000000000000 ) ) ;
#21096=CARTESIAN_POINT ( 'NONE',  ( -0.5626609578937310507, -0.5839878592448841665, -0.9562163583975410441 ) ) ;
#21126=EDGE_CURVE ( 'NONE', #9025, #11355, #19372, .T. ) ;
#21163=VECTOR ( 'NONE', #9985, 39.37007874015748143 ) ;
#21215=CARTESIAN_POINT ( 'NONE',  ( -0.1968503937007874127, -0.4724409448818898127, 0.8182917201112815953 ) ) ;
#21217=DIRECTION ( 'NONE',  ( 0.000000000000000000, 0.000000000000000000, 1.000000000000000000 ) ) ;
#21242=CIRCLE ( 'NONE', #16730, 0.6995255587571318490 ) ;
#21257=CIRCLE ( 'NONE', #1403, 1.131889763779527547 ) ;
#21281=DIRECTION ( 'NONE',  ( 0.000000000000000000, -1.000000000000000000, 0.000000000000000000 ) ) ;
#21286=DIRECTION ( 'NONE',  ( 1.000000000000000000, 0.000000000000000000, 0.000000000000000000 ) ) ;
#21324=ADVANCED_FACE ( 'NONE', ( #6409 ), #15341, .T. ) ;
#21343=CARTESIAN_POINT ( 'NONE',  ( -0.5761865902011245044, 1.104160307813825792, -0.07772139087856803907 ) ) ;
#21344=CARTESIAN_POINT ( 'NONE',  ( -0.1771653543307086520, 0.000000000000000000, 0.000000000000000000 ) ) ;
#21360=AXIS2_PLACEMENT_3D ( 'NONE', #3312, #9685, #22833 ) ;
#21361=DIRECTION ( 'NONE',  ( 0.000000000000000000, -1.000000000000000000, 0.000000000000000000 ) ) ;
#21388=AXIS2_PLACEMENT_3D ( 'NONE', #17222, #8742, #23994 ) ;
#21396=EDGE_CURVE ( 'NONE', #13772, #2222, #8539, .T. ) ;
#21424=CYLINDRICAL_SURFACE ( 'NONE', #8021, 0.8267716535433071723 ) ;
#21450=EDGE_CURVE ( 'NONE', #25692, #14534, #12987, .T. ) ;
#21457=AXIS2_PLACEMENT_3D ( 'NONE', #12595, #27860, #21217 ) ;
#21468=DIRECTION ( 'NONE',  ( -1.000000000000000000, 0.000000000000000000, 0.000000000000000000 ) ) ;
#21549=CYLINDRICAL_SURFACE ( 'NONE', #18985, 0.1082677165354330312 ) ;
#21555=DIRECTION ( 'NONE',  ( 0.000000000000000000, 1.000000000000000000, 0.000000000000000000 ) ) ;
#21606=CARTESIAN_POINT ( 'NONE',  ( -0.5616721359164329463, 1.121275077793840946, 0.01914631898357971665 ) ) ;
#21629=CIRCLE ( 'NONE', #15338, 0.1771653543307086798 ) ;
#21728=ORIENTED_EDGE ( 'NONE', *, *, #11372, .F. ) ;
#21731=AXIS2_PLACEMENT_3D ( 'NONE', #6461, #4599, #6744 ) ;
#21758=ADVANCED_FACE ( 'NONE', ( #20329 ), #8845, .F. ) ;
#21759=CARTESIAN_POINT ( 'NONE',  ( -0.5708661417322835607, 0.000000000000000000, 0.000000000000000000 ) ) ;
#21764=ORIENTED_EDGE ( 'NONE', *, *, #21126, .T. ) ;
#21779=CIRCLE ( 'NONE', #15040, 0.6889763779527560139 ) ;
#21786=LINE ( 'NONE', #4139, #2860 ) ;
#21805=CIRCLE ( 'NONE', #9600, 0.1771653543307086520 ) ;
#21808=CARTESIAN_POINT ( 'NONE',  ( -0.3661417322834645272, -0.4724409448818898127, 0.8182917201112815953 ) ) ;
#21816=AXIS2_PLACEMENT_3D ( 'NONE', #3024, #9116, #653 ) ;
#21821=EDGE_CURVE ( 'NONE', #23853, #3232, #19448, .T. ) ;
#21871=AXIS2_PLACEMENT_3D ( 'NONE', #12658, #18729, #10675 ) ;
#21896=DIRECTION ( 'NONE',  ( 0.000000000000000000, 1.000000000000000000, 0.000000000000000000 ) ) ;
#22014=CARTESIAN_POINT ( 'NONE',  ( -0.5738137315987272835, 1.106933345739570473, 0.07395176699327656034 ) ) ;
#22024=DIRECTION ( 'NONE',  ( -1.000000000000000000, 0.000000000000000000, 0.000000000000000000 ) ) ;
#22060=AXIS2_PLACEMENT_3D ( 'NONE', #16568, #5712, #21095 ) ;
#22105=EDGE_CURVE ( 'NONE', #5917, #11793, #6706, .T. ) ;
#22119=STYLED_ITEM ( 'NONE', ( #9484 ), #11975 ) ;
#22167=CARTESIAN_POINT ( 'NONE',  ( -0.3661417322834645272, -0.4724409448818898127, -0.8182917201112815953 ) ) ;
#22184=ORIENTED_EDGE ( 'NONE', *, *, #18470, .F. ) ;
#22195=EDGE_LOOP ( 'NONE', ( #7252, #7783 ) ) ;
#22203=ORIENTED_EDGE ( 'NONE', *, *, #12284, .F. ) ;
#22234=FACE_OUTER_BOUND ( 'NONE', #20165, .T. ) ;
#22248=ORIENTED_EDGE ( 'NONE', *, *, #3797, .F. ) ;
#22269=CLOSED_SHELL ( 'NONE', ( #21324, #21069, #18072, #15762, #22968, #19407, #11405, #22456, #4942, #24417, #6906, #22661, #20691, #13517, #21758, #24347, #4029, #19123, #22445, #16361, #20860, #20380, #20634, #24179, #9136, #25390, #20697, #17203, #24135, #7678, #16741, #7341, #4008, #2302, #15009, #2728, #13480, #25266, #6397, #18653, #19525, #2287, #7493 ) ) ;
#22300=ORIENTED_EDGE ( 'NONE', *, *, #21450, .T. ) ;
#22309=DIRECTION ( 'NONE',  ( 0.000000000000000000, -1.000000000000000000, 0.000000000000000000 ) ) ;
#22338=DIRECTION ( 'NONE',  ( 0.000000000000000000, -1.000000000000000000, 0.000000000000000000 ) ) ;
#22378=CARTESIAN_POINT ( 'NONE',  ( -0.5511811023622047445, 1.131889763744194921, -1.386165176156982434E-16 ) ) ;
#22382=CIRCLE ( 'NONE', #9753, 0.8267716535433071723 ) ;
#22409=VERTEX_POINT ( 'NONE', #9786 ) ;
#22411=VERTEX_POINT ( 'NONE', #18925 ) ;
#22436=CIRCLE ( 'NONE', #9344, 0.1082677165354330312 ) ;
#22445=ADVANCED_FACE ( 'NONE', ( #19209, #27838 ), #17636, .T. ) ;
#22456=ADVANCED_FACE ( 'NONE', ( #15412 ), #11143, .F. ) ;
#22458=CARTESIAN_POINT ( 'NONE',  ( -0.1771653543307086520, 0.8267716535433071723, 0.000000000000000000 ) ) ;
#22476=DIRECTION ( 'NONE',  ( 0.000000000000000000, 1.000000000000000000, 0.000000000000000000 ) ) ;
#22478=CIRCLE ( 'NONE', #7604, 0.1082677165354330728 ) ;
#22515=CYLINDRICAL_SURFACE ( 'NONE', #27034, 1.131889763779527547 ) ;
#22523=LINE ( 'NONE', #9938, #26984 ) ;
#22532=AXIS2_PLACEMENT_3D ( 'NONE', #1159, #17930, #22338 ) ;
#22551=VERTEX_POINT ( 'NONE', #26386 ) ;
#22554=EDGE_CURVE ( 'NONE', #26747, #16795, #1030, .T. ) ;
#22581=ORIENTED_EDGE ( 'NONE', *, *, #14071, .F. ) ;
#22597=ORIENTED_EDGE ( 'NONE', *, *, #3325, .F. ) ;
#22620=ORIENTED_EDGE ( 'NONE', *, *, #10189, .T. ) ;
#22653=CARTESIAN_POINT ( 'NONE',  ( -0.3937007874015748254, 0.000000000000000000, 0.000000000000000000 ) ) ;
#22655=FACE_OUTER_BOUND ( 'NONE', #23564, .T. ) ;
#22661=ADVANCED_FACE ( 'NONE', ( #25114 ), #24969, .F. ) ;
#22677=ORIENTED_EDGE ( 'NONE', *, *, #5327, .F. ) ;
#22689=VERTEX_POINT ( 'NONE', #18601 ) ;
#22696=DIRECTION ( 'NONE',  ( 0.000000000000000000, 0.000000000000000000, 1.000000000000000000 ) ) ;
#22699=AXIS2_PLACEMENT_3D ( 'NONE', #19563, #245, #4036 ) ;
#22716=ORIENTED_EDGE ( 'NONE', *, *, #9735, .F. ) ;
#22754=ORIENTED_EDGE ( 'NONE', *, *, #20927, .F. ) ;
#22761=LINE ( 'NONE', #20646, #19659 ) ;
#22773=ORIENTED_EDGE ( 'NONE', *, *, #27188, .F. ) ;
#22798=ORIENTED_EDGE ( 'NONE', *, *, #15270, .F. ) ;
#22813=CIRCLE ( 'NONE', #10153, 1.092519685039370136 ) ;
#22833=DIRECTION ( 'NONE',  ( 0.000000000000000000, -1.000000000000000000, 0.000000000000000000 ) ) ;
#22839=CARTESIAN_POINT ( 'NONE',  ( -0.2165354330708661457, 0.000000000000000000, 0.000000000000000000 ) ) ;
#22870=( NAMED_UNIT ( * ) SI_UNIT ( $, .STERADIAN. ) SOLID_ANGLE_UNIT ( ) ) ;
#22876=CARTESIAN_POINT ( 'NONE',  ( 2.664928230027803213, -0.4724409448818898127, 0.7100240035758484947 ) ) ;
#22882=DIRECTION ( 'NONE',  ( -1.000000000000000000, 0.000000000000000000, 0.000000000000000000 ) ) ;
#22896=ORIENTED_EDGE ( 'NONE', *, *, #11086, .T. ) ;
#22954=CIRCLE ( 'NONE', #25199, 0.1082677165354330312 ) ;
#22968=ADVANCED_FACE ( 'NONE', ( #15510 ), #5109, .T. ) ;
#22986=CARTESIAN_POINT ( 'NONE',  ( -0.5511811023622047445, 0.000000000000000000, 0.000000000000000000 ) ) ;
#23060=CARTESIAN_POINT ( 'NONE',  ( -0.3149606299212598381, 0.5905511811023621549, 0.000000000000000000 ) ) ;
#23086=CARTESIAN_POINT ( 'NONE',  ( -0.5656588455786464298, -0.5969388012308868285, -0.9446411342982088399 ) ) ;
#23100=EDGE_LOOP ( 'NONE', ( #7762, #16769, #16827, #7249 ) ) ;
#23109=ORIENTED_EDGE ( 'NONE', *, *, #20124, .T. ) ;
#23131=EDGE_CURVE ( 'NONE', #3232, #11793, #20858, .T. ) ;
#23146=ORIENTED_EDGE ( 'NONE', *, *, #17288, .T. ) ;
#23151=CARTESIAN_POINT ( 'NONE',  ( -0.02559055118110236185, 0.000000000000000000, 0.000000000000000000 ) ) ;
#23174=CARTESIAN_POINT ( 'NONE',  ( -0.3661417322834645272, 0.9448818897637796255, -1.639108661417322569E-17 ) ) ;
#23226=CARTESIAN_POINT ( 'NONE',  ( -0.5692984878077121946, -0.5056997808577781139, 0.9923580223634099751 ) ) ;
#23231=PLANE ( 'NONE',  #13996 ) ;
#23235=DIRECTION ( 'NONE',  ( 1.000000000000000000, 0.000000000000000000, 0.000000000000000000 ) ) ;
#23262=ORIENTED_EDGE ( 'NONE', *, *, #17412, .T. ) ;
#23264=FACE_BOUND ( 'NONE', #23355, .T. ) ;
#23309=CARTESIAN_POINT ( 'NONE',  ( -0.03937007874015747977, 0.000000000000000000, 0.000000000000000000 ) ) ;
#23316=EDGE_CURVE ( 'NONE', #16472, #16219, #8519, .T. ) ;
#23355=EDGE_LOOP ( 'NONE', ( #8351, #15891 ) ) ;
#23356=CARTESIAN_POINT ( 'NONE',  ( -0.5905511811023621549, 1.087444635826771533, 0.1051828227901525498 ) ) ;
#23375=CARTESIAN_POINT ( 'NONE',  ( -0.5811915241081616612, -0.4724399524670138684, 0.9954595399565421276 ) ) ;
#23379=CARTESIAN_POINT ( 'NONE',  ( -0.5744830435817726011, -0.4891464190265612522, -0.9948699164926496641 ) ) ;
#23388=EDGE_CURVE ( 'NONE', #27836, #12685, #844, .T. ) ;
#23417=CONICAL_SURFACE ( 'NONE', #11661, 0.6102362204724409711, 0.7853981625000032718 ) ;
#23446=VERTEX_POINT ( 'NONE', #11032 ) ;
#23452=EDGE_LOOP ( 'NONE', ( #20424, #5927, #20069, #22754 ) ) ;
#23477=CIRCLE ( 'NONE', #15786, 0.5905511811023621549 ) ;
#23490=EDGE_LOOP ( 'NONE', ( #10498, #903 ) ) ;
#23545=EDGE_LOOP ( 'NONE', ( #16779, #8640, #18746, #19353 ) ) ;
#23547=DIRECTION ( 'NONE',  ( 0.000000000000000000, 0.000000000000000000, 1.000000000000000000 ) ) ;
#23564=EDGE_LOOP ( 'NONE', ( #828, #6484, #4275, #26775 ) ) ;
#23592=DIRECTION ( 'NONE',  ( 0.000000000000000000, 0.000000000000000000, 1.000000000000000000 ) ) ;
#23615=LINE ( 'NONE', #2528, #3516 ) ;
#23638=AXIS2_PLACEMENT_3D ( 'NONE', #2512, #9846, #18445 ) ;
#23649=DIRECTION ( 'NONE',  ( 0.000000000000000000, -1.000000000000000000, 0.000000000000000000 ) ) ;
#23661=EDGE_CURVE ( 'NONE', #14534, #5538, #14273, .T. ) ;
#23663=VERTEX_POINT ( 'NONE', #10020 ) ;
#23674=DIRECTION ( 'NONE',  ( -1.000000000000000000, 0.000000000000000000, 0.000000000000000000 ) ) ;
#23723=ORIENTED_EDGE ( 'NONE', *, *, #27274, .T. ) ;
#23729=EDGE_LOOP ( 'NONE', ( #4384, #10866 ) ) ;
#23747=CARTESIAN_POINT ( 'NONE',  ( -0.5610236220428271858, 1.122047244090071949, 1.311930826979132746E-15 ) ) ;
#23786=DIRECTION ( 'NONE',  ( -1.000000000000000000, 0.000000000000000000, 0.000000000000000000 ) ) ;
#23792=LINE ( 'NONE', #2438, #6684 ) ;
#23794=DIRECTION ( 'NONE',  ( 0.000000000000000000, -1.000000000000000000, 0.000000000000000000 ) ) ;
#23800=CARTESIAN_POINT ( 'NONE',  ( -0.3661417322834645272, -0.4724409448818898127, 0.8182917201112815953 ) ) ;
#23821=DIRECTION ( 'NONE',  ( 0.000000000000000000, -1.000000000000000000, 0.000000000000000000 ) ) ;
#23845=ORIENTED_EDGE ( 'NONE', *, *, #10581, .T. ) ;
#23853=VERTEX_POINT ( 'NONE', #20155 ) ;
#23859=ORIENTED_EDGE ( 'NONE', *, *, #22554, .F. ) ;
#23884=PLANE ( 'NONE',  #13386 ) ;
#23892=AXIS2_PLACEMENT_3D ( 'NONE', #25794, #12656, #23821 ) ;
#23914=AXIS2_PLACEMENT_3D ( 'NONE', #7182, #22024, #13670 ) ;
#23947=VECTOR ( 'NONE', #27075, 39.37007874015748143 ) ;
#23977=CARTESIAN_POINT ( 'NONE',  ( -2.185478346456693112E-16, 0.000000000000000000, 0.000000000000000000 ) ) ;
#23994=DIRECTION ( 'NONE',  ( 0.000000000000000000, 1.000000000000000000, 0.000000000000000000 ) ) ;
#24035=AXIS2_PLACEMENT_3D ( 'NONE', #27725, #4127, #21361 ) ;
#24121=AXIS2_PLACEMENT_3D ( 'NONE', #2114, #19203, #14580 ) ;
#24135=ADVANCED_FACE ( 'NONE', ( #5654 ), #18910, .F. ) ;
#24161=AXIS2_PLACEMENT_3D ( 'NONE', #6815, #13568, #2687 ) ;
#24179=ADVANCED_FACE ( 'NONE', ( #6084, #1548 ), #1402, .T. ) ;
#24181=DIRECTION ( 'NONE',  ( 0.000000000000000000, 1.000000000000000000, 0.000000000000000000 ) ) ;
#24184=CARTESIAN_POINT ( 'NONE',  ( -0.5905511811023621549, -0.4724409448818898127, 0.6411263657805729155 ) ) ;
#24227=DIRECTION ( 'NONE',  ( 0.000000000000000000, 0.000000000000000000, 1.000000000000000000 ) ) ;
#24237=EDGE_CURVE ( 'NONE', #8838, #27393, #21786, .T. ) ;
#24241=DIRECTION ( 'NONE',  ( 0.000000000000000000, -1.000000000000000000, 0.000000000000000000 ) ) ;
#24267=AXIS2_PLACEMENT_3D ( 'NONE', #3124, #9624, #14022 ) ;
#24271=DIRECTION ( 'NONE',  ( -1.000000000000000000, 0.000000000000000000, 0.000000000000000000 ) ) ;
#24299=AXIS2_PLACEMENT_3D ( 'NONE', #21759, #4248, #11018 ) ;
#24323=EDGE_CURVE ( 'NONE', #17036, #9597, #25221, .T. ) ;
#24347=ADVANCED_FACE ( 'NONE', ( #22234 ), #2859, .T. ) ;
#24362=EDGE_CURVE ( 'NONE', #18929, #3892, #16304, .T. ) ;
#24372=COLOUR_RGB ( '', 0.08235294, 0.09019608, 0.10196078) ;
#24417=ADVANCED_FACE ( 'NONE', ( #22655 ), #18537, .F. ) ;
#24424=EDGE_CURVE ( 'NONE', #12685, #10034, #10532, .T. ) ;
#24551=ORIENTED_EDGE ( 'NONE', *, *, #12405, .T. ) ;
#24652=ORIENTED_EDGE ( 'NONE', *, *, #20995, .F. ) ;
#24710=CARTESIAN_POINT ( 'NONE',  ( -0.4783464566929133688, -0.4724409448818898127, 0.8182917201112815953 ) ) ;
#24798=ORIENTED_EDGE ( 'NONE', *, *, #12284, .T. ) ;
#24818=MECHANICAL_DESIGN_GEOMETRIC_PRESENTATION_REPRESENTATION('',(#22119),#6791);
#24828=ORIENTED_EDGE ( 'NONE', *, *, #11571, .T. ) ;
#24891=FILL_AREA_STYLE ('',( #7812 ) ) ;
#24906=DIRECTION ( 'NONE',  ( 0.000000000000000000, 1.000000000000000000, 0.000000000000000000 ) ) ;
#24922=EDGE_LOOP ( 'NONE', ( #17513, #20638, #3897, #5774 ) ) ;
#24951=VECTOR ( 'NONE', #19810, 39.37007874015748143 ) ;
#24953=CARTESIAN_POINT ( 'NONE',  ( -0.3661417322834645272, -0.4724409448818898127, -0.7100240035758484947 ) ) ;
#24969=CYLINDRICAL_SURFACE ( 'NONE', #6926, 0.1082677165354330728 ) ;
#25049=ORIENTED_EDGE ( 'NONE', *, *, #25590, .T. ) ;
#25114=FACE_OUTER_BOUND ( 'NONE', #3357, .T. ) ;
#25115=( LENGTH_UNIT ( ) NAMED_UNIT ( * ) SI_UNIT ( $, .METRE. ) ) ;
#25118=FACE_OUTER_BOUND ( 'NONE', #17705, .T. ) ;
#25199=AXIS2_PLACEMENT_3D ( 'NONE', #2363, #4622, #23592 ) ;
#25206=CIRCLE ( 'NONE', #12577, 0.8267716535433071723 ) ;
#25217=EDGE_CURVE ( 'NONE', #11793, #3232, #15132, .T. ) ;
#25220=LINE ( 'NONE', #5890, #2549 ) ;
#25221=LINE ( 'NONE', #18852, #8305 ) ;
#25260=ORIENTED_EDGE ( 'NONE', *, *, #9443, .T. ) ;
#25266=ADVANCED_FACE ( 'NONE', ( #4190 ), #6036, .F. ) ;
#25298=ORIENTED_EDGE ( 'NONE', *, *, #19338, .T. ) ;
#25326=CARTESIAN_POINT ( 'NONE',  ( -0.5776041937077627253, -0.4807970751194731163, -0.9954635886629241703 ) ) ;
#25334=DIRECTION ( 'NONE',  ( 1.000000000000000000, 0.000000000000000000, 0.000000000000000000 ) ) ;
#25351=EDGE_LOOP ( 'NONE', ( #13786, #18736 ) ) ;
#25353=DIRECTION ( 'NONE',  ( 1.000000000000000000, 0.000000000000000000, 0.000000000000000000 ) ) ;
#25356=PRODUCT ( 'Rear Bearing Cover', 'Rear Bearing Cover', '', ( #8437 ) ) ;
#25390=ADVANCED_FACE ( 'NONE', ( #11095 ), #2904, .T. ) ;
#25413=ORIENTED_EDGE ( 'NONE', *, *, #11831, .F. ) ;
#25416=VERTEX_POINT ( 'NONE', #4463 ) ;
#25418=AXIS2_PLACEMENT_3D ( 'NONE', #19371, #10893, #6664 ) ;
#25440=ORIENTED_EDGE ( 'NONE', *, *, #25762, .F. ) ;
#25475=CARTESIAN_POINT ( 'NONE',  ( -0.5751341951449447931, -0.6192718686200742173, 0.9188498711508340522 ) ) ;
#25480=CARTESIAN_POINT ( 'NONE',  ( -0.5670365097597637183, -0.5142378326786118947, -0.9905099408301584196 ) ) ;
#25505=FACE_OUTER_BOUND ( 'NONE', #25351, .T. ) ;
#25516=EDGE_CURVE ( 'NONE', #18462, #5530, #10140, .T. ) ;
#25517=AXIS2_PLACEMENT_3D ( 'NONE', #14552, #14258, #26960 ) ;
#25525=CARTESIAN_POINT ( 'NONE',  ( -0.5840206614248149020, -0.4658374228744227574, -0.9954608982700227093 ) ) ;
#25536=CARTESIAN_POINT ( 'NONE',  ( -0.4783464566929133688, -0.4724409448818898127, -0.9954570744419902750 ) ) ;
#25537=VERTEX_POINT ( 'NONE', #7656 ) ;
#25555=CYLINDRICAL_SURFACE ( 'NONE', #5446, 0.1771653543307086798 ) ;
#25571=CARTESIAN_POINT ( 'NONE',  ( -0.5905511811023621549, 0.000000000000000000, 0.000000000000000000 ) ) ;
#25581=CARTESIAN_POINT ( 'NONE',  ( 2.664928230027803213, 0.9448818897637796255, -1.639108661417322569E-17 ) ) ;
#25590=EDGE_CURVE ( 'NONE', #16095, #218, #22761, .T. ) ;
#25597=DIRECTION ( 'NONE',  ( 0.000000000000000000, -1.000000000000000000, 0.000000000000000000 ) ) ;
#25649=CARTESIAN_POINT ( 'NONE',  ( -0.3661417322834645272, -0.4724409448818898127, 0.8182917201112815953 ) ) ;
#25655=EDGE_CURVE ( 'NONE', #18321, #17036, #18726, .T. ) ;
#25663=CARTESIAN_POINT ( 'NONE',  ( -0.5871411979517291435, -0.4592307444200218747, -0.9950886577925481813 ) ) ;
#25664=VECTOR ( 'NONE', #6576, 39.37007874015748143 ) ;
#25692=VERTEX_POINT ( 'NONE', #23356 ) ;
#25720=CYLINDRICAL_SURFACE ( 'NONE', #8086, 0.1082677165354330728 ) ;
#25759=DIRECTION ( 'NONE',  ( 0.000000000000000000, -1.000000000000000000, 0.000000000000000000 ) ) ;
#25761=VERTEX_POINT ( 'NONE', #20336 ) ;
#25762=EDGE_CURVE ( 'NONE', #27393, #3892, #1143, .T. ) ;
#25780=CYLINDRICAL_SURFACE ( 'NONE', #20560, 1.131889763779527547 ) ;
#25794=CARTESIAN_POINT ( 'NONE',  ( -0.5511811023622047445, 0.000000000000000000, 0.000000000000000000 ) ) ;
#25806=ORIENTED_EDGE ( 'NONE', *, *, #20927, .T. ) ;
#25842=CARTESIAN_POINT ( 'NONE',  ( -0.5905511811023621549, 1.087444635826771533, 0.1051828227901525498 ) ) ;
#25843=CARTESIAN_POINT ( 'NONE',  ( -0.2362204724409449064, 1.131889763779527547, 0.000000000000000000 ) ) ;
#25900=EDGE_CURVE ( 'NONE', #10034, #22689, #16187, .T. ) ;
#25946=CARTESIAN_POINT ( 'NONE',  ( -0.1968503937007874127, 0.9448818897637796255, -1.639108661417322569E-17 ) ) ;
#25962=EDGE_LOOP ( 'NONE', ( #27561, #6992, #11913, #1005, #20914, #18361, #5578, #5746 ) ) ;
#26019=EDGE_LOOP ( 'NONE', ( #16698, #16247, #25806, #5283 ) ) ;
#26023=CIRCLE ( 'NONE', #14296, 0.5905511811023621549 ) ;
#26026=CARTESIAN_POINT ( 'NONE',  ( -0.1771653543307086520, 0.000000000000000000, 0.000000000000000000 ) ) ;
#26075=CIRCLE ( 'NONE', #2610, 0.1771653543307086520 ) ;
#26103=DIRECTION ( 'NONE',  ( 0.000000000000000000, 0.000000000000000000, 1.000000000000000000 ) ) ;
#26106=VECTOR ( 'NONE', #19936, 39.37007874015748143 ) ;
#26168=CIRCLE ( 'NONE', #14456, 0.1771653543307086798 ) ;
#26264=FACE_BOUND ( 'NONE', #9430, .T. ) ;
#26294=ORIENTED_EDGE ( 'NONE', *, *, #9817, .T. ) ;
#26296=DIRECTION ( 'NONE',  ( 1.000000000000000000, 0.000000000000000000, 0.000000000000000000 ) ) ;
#26331=CARTESIAN_POINT ( 'NONE',  ( -0.1574803149606299191, 0.5905511811023621549, 0.000000000000000000 ) ) ;
#26362=CARTESIAN_POINT ( 'NONE',  ( -0.4783464566929133688, 0.9448818897637796255, 0.1771653543307086520 ) ) ;
#26371=DIRECTION ( 'NONE',  ( 1.000000000000000000, 0.000000000000000000, 0.000000000000000000 ) ) ;
#26386=CARTESIAN_POINT ( 'NONE',  ( -0.1968503937007874127, 0.8267716535433071723, 0.000000000000000000 ) ) ;
#26403=CARTESIAN_POINT ( 'NONE',  ( -0.3661417322834645272, -0.4724409448818898127, 0.7100240035758484947 ) ) ;
#26409=ORIENTED_EDGE ( 'NONE', *, *, #24362, .T. ) ;
#26421=CARTESIAN_POINT ( 'NONE',  ( -0.1968503937007874127, 0.000000000000000000, 0.000000000000000000 ) ) ;
#26423=CYLINDRICAL_SURFACE ( 'NONE', #13014, 0.8267716535433071723 ) ;
#26481=EDGE_CURVE ( 'NONE', #22551, #12001, #4751, .T. ) ;
#26483=ORIENTED_EDGE ( 'NONE', *, *, #18470, .T. ) ;
#26496=PRODUCT_DEFINITION_FORMATION_WITH_SPECIFIED_SOURCE ( 'ANY', '', #25356, .NOT_KNOWN. ) ;
#26514=ORIENTED_EDGE ( 'NONE', *, *, #27124, .F. ) ;
#26548=EDGE_CURVE ( 'NONE', #16795, #26747, #9251, .T. ) ;
#26564=CARTESIAN_POINT ( 'NONE',  ( -0.1968503937007874127, -0.4724409448818898127, -0.8182917201112815953 ) ) ;
#26603=DIRECTION ( 'NONE',  ( 0.000000000000000000, 0.000000000000000000, 1.000000000000000000 ) ) ;
#26645=CIRCLE ( 'NONE', #11312, 0.1082677165354330728 ) ;
#26662=LENGTH_MEASURE_WITH_UNIT ( LENGTH_MEASURE( 0.02539999999999999897 ), #25115 ) ;
#26702=ORIENTED_EDGE ( 'NONE', *, *, #5981, .F. ) ;
#26709=EDGE_CURVE ( 'NONE', #8922, #13827, #22382, .T. ) ;
#26714=CARTESIAN_POINT ( 'NONE',  ( -0.1771653543307086520, -0.7539370078740157410, 9.233065434516462138E-17 ) ) ;
#26719=CYLINDRICAL_SURFACE ( 'NONE', #24267, 0.1771653543307086798 ) ;
#26723=LENGTH_MEASURE_WITH_UNIT ( LENGTH_MEASURE( 0.02539999999999999897 ), #18372 ) ;
#26729=ORIENTED_EDGE ( 'NONE', *, *, #18002, .F. ) ;
#26740=FACE_OUTER_BOUND ( 'NONE', #14750, .T. ) ;
#26747=VERTEX_POINT ( 'NONE', #26844 ) ;
#26758=AXIS2_PLACEMENT_3D ( 'NONE', #7019, #15641, #24241 ) ;
#26775=ORIENTED_EDGE ( 'NONE', *, *, #24362, .F. ) ;
#26820=EDGE_CURVE ( 'NONE', #14042, #23853, #27246, .T. ) ;
#26844=CARTESIAN_POINT ( 'NONE',  ( -2.185478346456693112E-16, -0.8162224727389330026, 0.000000000000000000 ) ) ;
#26879=AXIS2_PLACEMENT_3D ( 'NONE', #23151, #1254, #18459 ) ;
#26889=CARTESIAN_POINT ( 'NONE',  ( 2.664928230027803213, -0.4724409448818898127, -0.7100240035758484947 ) ) ;
#26921=CIRCLE ( 'NONE', #15207, 0.8267716535433071723 ) ;
#26933=ORIENTED_EDGE ( 'NONE', *, *, #3133, .F. ) ;
#26960=DIRECTION ( 'NONE',  ( 0.000000000000000000, 1.000000000000000000, 0.000000000000000000 ) ) ;
#26969=CIRCLE ( 'NONE', #10255, 0.7539370078740157410 ) ;
#26984=VECTOR ( 'NONE', #16310, 39.37007874015748143 ) ;
#27025=CARTESIAN_POINT ( 'NONE',  ( -0.1968503937007874127, -0.8267716535433071723, 1.012503259137575512E-16 ) ) ;
#27034=AXIS2_PLACEMENT_3D ( 'NONE', #22653, #912, #5275 ) ;
#27038=DIRECTION ( 'NONE',  ( 1.000000000000000000, 0.000000000000000000, 0.000000000000000000 ) ) ;
#27046=ORIENTED_EDGE ( 'NONE', *, *, #11001, .T. ) ;
#27075=DIRECTION ( 'NONE',  ( 1.000000000000000000, 0.000000000000000000, 0.000000000000000000 ) ) ;
#27106=( CONVERSION_BASED_UNIT ( 'INCH', #26662 ) LENGTH_UNIT ( ) NAMED_UNIT ( #13586 ) ) ;
#27124=EDGE_CURVE ( 'NONE', #3293, #9025, #5638, .T. ) ;
#27126=UNCERTAINTY_MEASURE_WITH_UNIT (LENGTH_MEASURE( 1.000000000000000082E-05 ), #27106, 'distance_accuracy_value', 'NONE') ;
#27140=ORIENTED_EDGE ( 'NONE', *, *, #23316, .T. ) ;
#27184=DIRECTION ( 'NONE',  ( -1.000000000000000000, 0.000000000000000000, 0.000000000000000000 ) ) ;
#27188=EDGE_CURVE ( 'NONE', #22411, #14218, #26921, .T. ) ;
#27195=VERTEX_POINT ( 'NONE', #10421 ) ;
#27246=B_SPLINE_CURVE_WITH_KNOTS ( 'NONE', 3,
 ( #8617, #16828, #19354, #21343, #6649, #8756, #12989, #19488, #15275, #15136, #23747 ),
 .UNSPECIFIED., .F., .F.,
 ( 4, 2, 1, 2, 2, 4 ),
 ( 0.000000000000000000, 0.1249999999999981681, 0.1874999999999971689, 0.2187499999999970024, 0.2499999999999968359, 0.5000000000000000000 ),
 .UNSPECIFIED. ) ;
#27274=EDGE_CURVE ( 'NONE', #17602, #19029, #1655, .T. ) ;
#27291=FACE_OUTER_BOUND ( 'NONE', #9387, .T. ) ;
#27300=EDGE_CURVE ( 'NONE', #1935, #25537, #25220, .T. ) ;
#27393=VERTEX_POINT ( 'NONE', #6855 ) ;
#27394=EDGE_LOOP ( 'NONE', ( #14764, #27849, #16590, #19333 ) ) ;
#27399=DIRECTION ( 'NONE',  ( 0.000000000000000000, 1.000000000000000000, 0.000000000000000000 ) ) ;
#27413=ORIENTED_EDGE ( 'NONE', *, *, #21126, .F. ) ;
#27455=CARTESIAN_POINT ( 'NONE',  ( -0.5656587879800142327, -0.5969381639805851902, 0.9446416071465162378 ) ) ;
#27497=DIRECTION ( 'NONE',  ( -1.000000000000000000, 0.000000000000000000, 0.000000000000000000 ) ) ;
#27511=DIRECTION ( 'NONE',  ( -1.000000000000000000, 0.000000000000000000, 0.000000000000000000 ) ) ;
#27541=AXIS2_PLACEMENT_3D ( 'NONE', #3942, #5931, #8327 ) ;
#27548=ORIENTED_EDGE ( 'NONE', *, *, #14157, .F. ) ;
#27550=ADVANCED_BREP_SHAPE_REPRESENTATION ( 'Rear Bearing Cover', ( #11975, #11588 ), #19278 ) ;
#27561=ORIENTED_EDGE ( 'NONE', *, *, #26820, .T. ) ;
#27606=CARTESIAN_POINT ( 'NONE',  ( -0.3661417322834645272, 0.9448818897637796255, -1.639108661417322569E-17 ) ) ;
#27612=DIRECTION ( 'NONE',  ( -0.9659258263664933786, -0.2588190448135661570, 0.000000000000000000 ) ) ;
#27681=CIRCLE ( 'NONE', #19979, 1.092519685039370136 ) ;
#27705=FACE_OUTER_BOUND ( 'NONE', #10557, .T. ) ;
#27706=AXIS2_PLACEMENT_3D ( 'NONE', #14278, #21038, #12280 ) ;
#27725=CARTESIAN_POINT ( 'NONE',  ( -0.01968503937007897581, 0.000000000000000000, 0.000000000000000000 ) ) ;
#27734=EDGE_CURVE ( 'NONE', #22409, #10034, #14824, .T. ) ;
#27754=ORIENTED_EDGE ( 'NONE', *, *, #23661, .T. ) ;
#27760=ORIENTED_EDGE ( 'NONE', *, *, #17780, .T. ) ;
#27761=AXIS2_PLACEMENT_3D ( 'NONE', #3534, #7940, #1430 ) ;
#27767=FACE_BOUND ( 'NONE', #15282, .T. ) ;
#27812=ORIENTED_EDGE ( 'NONE', *, *, #4650, .T. ) ;
#27816=VERTEX_POINT ( 'NONE', #16777 ) ;
#27836=VERTEX_POINT ( 'NONE', #7639 ) ;
#27838=FACE_OUTER_BOUND ( 'NONE', #15707, .T. ) ;
#27849=ORIENTED_EDGE ( 'NONE', *, *, #23131, .F. ) ;
#27860=DIRECTION ( 'NONE',  ( -1.000000000000000000, 0.000000000000000000, 0.000000000000000000 ) ) ;
#27873=EDGE_CURVE ( 'NONE', #23663, #9597, #19723, .T. ) ;
ENDSEC;
END-ISO-10303-21;
